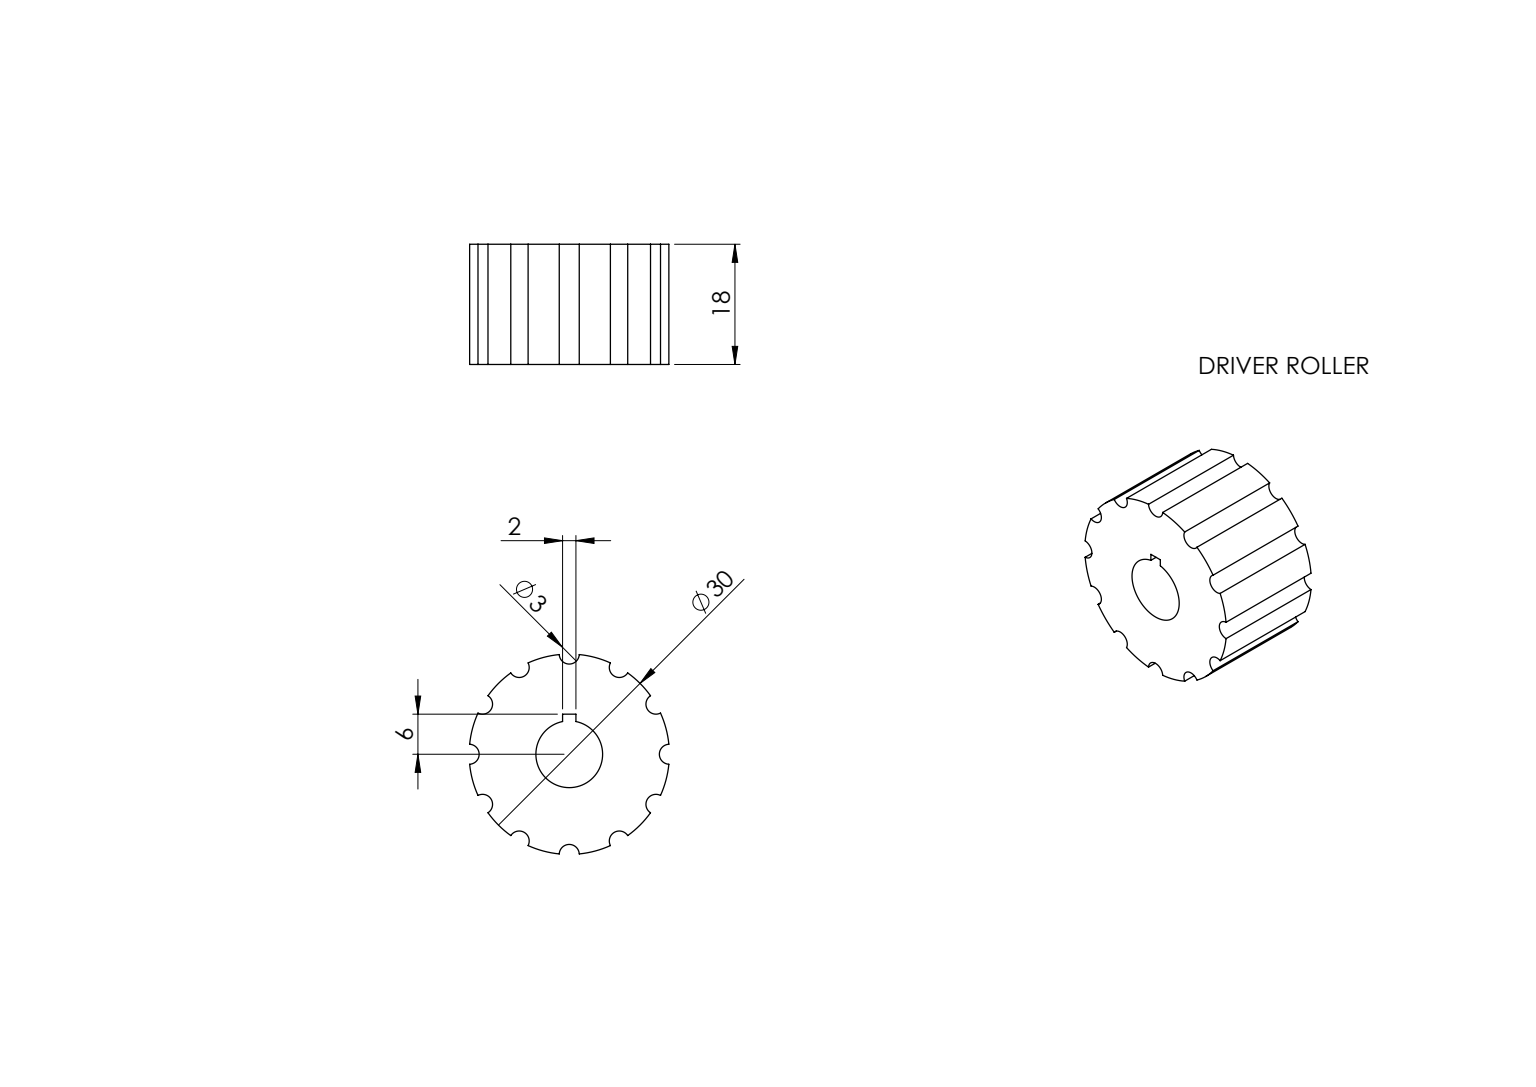
ISO-10303-21;
HEADER;
FILE_DESCRIPTION (('STEP AP214'),
    '1' );
FILE_NAME ('driver roller.step',
    '2026-10-25T07:12:54',
    ( '' ),
    ( '' ),
    'SwSTEP 2.0',
    'SolidWorks 2026',
    '' );
FILE_SCHEMA (( 'AUTOMOTIVE_DESIGN' ));
ENDSEC;

DATA;
#4=DIRECTION ( 'NONE',  ( 0.4999999999999977796, 0.8660254037844398178, 0.000000000000000000 ) ) ;
#12=AXIS2_PLACEMENT_3D ( 'NONE', #12108, #3741, #674 ) ;
#15=CARTESIAN_POINT ( 'NONE',  ( 2.449293598294706513E-15, -35.00000000000000000, 9.000000000000000000 ) ) ;
#19=ADVANCED_FACE ( 'NONE', ( #12392 ), #1035, .T. ) ;
#25=DIRECTION ( 'NONE',  ( -0.000000000000000000, -0.000000000000000000, 1.000000000000000000 ) ) ;
#49=VECTOR ( 'NONE', #8618, 1000.000000000000000 ) ;
#66=CIRCLE ( 'NONE', #7586, 1.500000000000001110 ) ;
#68=LINE ( 'NONE', #4288, #2309 ) ;
#80=CYLINDRICAL_SURFACE ( 'NONE', #13518, 1.500000000000001332 ) ;
#102=DIRECTION ( 'NONE',  ( 1.000000000000000000, 0.000000000000000000, 0.000000000000000000 ) ) ;
#120=ADVANCED_FACE ( 'NONE', ( #5352 ), #80, .F. ) ;
#146=ORIENTED_EDGE ( 'NONE', *, *, #5916, .F. ) ;
#151=DIRECTION ( 'NONE',  ( -0.5000000000000041078, 0.8660254037844362651, 0.000000000000000000 ) ) ;
#153=FACE_OUTER_BOUND ( 'NONE', #3940, .T. ) ;
#154=FACE_OUTER_BOUND ( 'NONE', #10455, .T. ) ;
#193=CYLINDRICAL_SURFACE ( 'NONE', #11066, 15.00000000000000000 ) ;
#198=ORIENTED_EDGE ( 'NONE', *, *, #8722, .T. ) ;
#201=CIRCLE ( 'NONE', #9264, 1.500000000000000222 ) ;
#208=CARTESIAN_POINT ( 'NONE',  ( 2.449293598294706513E-15, -20.00000000000000000, -9.000000000000000000 ) ) ;
#213=ORIENTED_EDGE ( 'NONE', *, *, #10321, .T. ) ;
#227=EDGE_CURVE ( 'NONE', #4104, #6571, #11764, .T. ) ;
#231=VECTOR ( 'NONE', #11750, 1000.000000000000000 ) ;
#239=CARTESIAN_POINT ( 'NONE',  ( 2.449293598294706513E-15, -20.00000000000000000, 9.000000000000000000 ) ) ;
#261=ORIENTED_EDGE ( 'NONE', *, *, #227, .F. ) ;
#265=CARTESIAN_POINT ( 'NONE',  ( 2.449293598294706513E-15, -20.00000000000000000, 9.000000000000000000 ) ) ;
#272=EDGE_CURVE ( 'NONE', #12293, #940, #9194, .T. ) ;
#276=AXIS2_PLACEMENT_3D ( 'NONE', #9355, #962, #6117 ) ;
#277=ORIENTED_EDGE ( 'NONE', *, *, #8722, .F. ) ;
#278=VERTEX_POINT ( 'NONE', #10857 ) ;
#297=ADVANCED_FACE ( 'NONE', ( #10786 ), #7829, .T. ) ;
#299=DIRECTION ( 'NONE',  ( -0.000000000000000000, -0.000000000000000000, -1.000000000000000000 ) ) ;
#310=CIRCLE ( 'NONE', #5415, 1.499999999999999778 ) ;
#317=DIRECTION ( 'NONE',  ( -0.000000000000000000, -0.000000000000000000, 1.000000000000000000 ) ) ;
#318=( NAMED_UNIT ( * ) PLANE_ANGLE_UNIT ( ) SI_UNIT ( $, .RADIAN. ) );
#335=CARTESIAN_POINT ( 'NONE',  ( -11.49038105676659249, -12.50000000000003020, -9.000000000000000000 ) ) ;
#344=ORIENTED_EDGE ( 'NONE', *, *, #1521, .T. ) ;
#348=AXIS2_PLACEMENT_3D ( 'NONE', #13063, #10988, #12044 ) ;
#349=DIRECTION ( 'NONE',  ( 1.000000000000000000, 0.000000000000000000, 0.000000000000000000 ) ) ;
#375=ORIENTED_EDGE ( 'NONE', *, *, #2646, .F. ) ;
#392=ORIENTED_EDGE ( 'NONE', *, *, #1283, .T. ) ;
#402=CARTESIAN_POINT ( 'NONE',  ( 13.67449106481161003, -13.83491329190030861, 9.000000000000000000 ) ) ;
#411=DIRECTION ( 'NONE',  ( -0.000000000000000000, -0.000000000000000000, -1.000000000000000000 ) ) ;
#415=CARTESIAN_POINT ( 'NONE',  ( -6.165086708099452473, -33.67449106481171128, 9.000000000000000000 ) ) ;
#416=CARTESIAN_POINT ( 'NONE',  ( 14.92500000000001492, -21.49812382665770727, -9.000000000000000000 ) ) ;
#430=AXIS2_PLACEMENT_3D ( 'NONE', #5828, #10990, #3471 ) ;
#439=VERTEX_POINT ( 'NONE', #5171 ) ;
#442=CARTESIAN_POINT ( 'NONE',  ( 2.449293598294706513E-15, -20.00000000000000000, 9.000000000000000000 ) ) ;
#453=CIRCLE ( 'NONE', #6010, 5.000000000000000888 ) ;
#476=DIRECTION ( 'NONE',  ( -1.000000000000000000, 0.000000000000000000, 0.000000000000000000 ) ) ;
#478=CARTESIAN_POINT ( 'NONE',  ( -0.9999999999999976685, -20.00000000000000000, 8.999999999999998224 ) ) ;
#483=DIRECTION ( 'NONE',  ( -1.000000000000000000, 0.000000000000000000, 0.000000000000000000 ) ) ;
#487=CARTESIAN_POINT ( 'NONE',  ( 1.000000000000000000, -14.00000000000000000, 8.999999999999998224 ) ) ;
#505=EDGE_CURVE ( 'NONE', #7167, #13447, #11471, .T. ) ;
#535=ORIENTED_EDGE ( 'NONE', *, *, #11080, .F. ) ;
#543=LINE ( 'NONE', #8998, #5245 ) ;
#552=EDGE_LOOP ( 'NONE', ( #11570, #2557, #1287, #708 ) ) ;
#554=CARTESIAN_POINT ( 'NONE',  ( 2.449293598294706513E-15, -20.00000000000000000, 9.000000000000000000 ) ) ;
#561=CARTESIAN_POINT ( 'NONE',  ( -1.498123826657861590, -5.075000000000000178, 9.000000000000000000 ) ) ;
#569=DIRECTION ( 'NONE',  ( 1.000000000000000000, 0.000000000000000000, 0.000000000000000000 ) ) ;
#575=LINE ( 'NONE', #4688, #3098 ) ;
#579=VERTEX_POINT ( 'NONE', #9306 ) ;
#580=ORIENTED_EDGE ( 'NONE', *, *, #12965, .T. ) ;
#582=VERTEX_POINT ( 'NONE', #4050 ) ;
#585=EDGE_CURVE ( 'NONE', #579, #13009, #3012, .T. ) ;
#613=ORIENTED_EDGE ( 'NONE', *, *, #4413, .T. ) ;
#625=DIRECTION ( 'NONE',  ( 1.000000000000000000, 0.000000000000000000, 0.000000000000000000 ) ) ;
#631=CARTESIAN_POINT ( 'NONE',  ( 13.67449106481173615, -26.16508670809940895, 0.000000000000000000 ) ) ;
#636=DIRECTION ( 'NONE',  ( 0.000000000000000000, 0.000000000000000000, -1.000000000000000000 ) ) ;
#655=LINE ( 'NONE', #4833, #12685 ) ;
#672=DIRECTION ( 'NONE',  ( -0.000000000000000000, 0.000000000000000000, 1.000000000000000000 ) ) ;
#674=DIRECTION ( 'NONE',  ( 0.4999999999999977796, 0.8660254037844398178, 0.000000000000000000 ) ) ;
#689=EDGE_CURVE ( 'NONE', #12154, #1369, #11986, .T. ) ;
#694=CARTESIAN_POINT ( 'NONE',  ( -14.92499999999998828, -21.49812382665792754, -9.000000000000000000 ) ) ;
#704=CARTESIAN_POINT ( 'NONE',  ( 6.165086708099353885, -6.325508935188239867, -9.000000000000000000 ) ) ;
#708=ORIENTED_EDGE ( 'NONE', *, *, #3659, .T. ) ;
#744=CYLINDRICAL_SURFACE ( 'NONE', #7474, 1.500000000000001332 ) ;
#746=AXIS2_PLACEMENT_3D ( 'NONE', #10700, #7661, #9662 ) ;
#758=EDGE_LOOP ( 'NONE', ( #6496, #10523, #13430, #10250 ) ) ;
#761=ORIENTED_EDGE ( 'NONE', *, *, #9825, .T. ) ;
#762=EDGE_LOOP ( 'NONE', ( #12304, #11458, #12169, #8097 ) ) ;
#769=EDGE_CURVE ( 'NONE', #9673, #2278, #201, .T. ) ;
#772=CARTESIAN_POINT ( 'NONE',  ( -12.99038105676654453, -27.50000000000006040, -9.000000000000000000 ) ) ;
#796=ORIENTED_EDGE ( 'NONE', *, *, #2151, .F. ) ;
#803=CARTESIAN_POINT ( 'NONE',  ( -13.49999999999999467, -20.00000000000005329, 9.000000000000000000 ) ) ;
#807=ORIENTED_EDGE ( 'NONE', *, *, #11080, .T. ) ;
#812=CARTESIAN_POINT ( 'NONE',  ( 8.759913291900563337, -32.17636723815374467, 9.000000000000000000 ) ) ;
#821=ORIENTED_EDGE ( 'NONE', *, *, #11191, .T. ) ;
#825=DIRECTION ( 'NONE',  ( -0.000000000000000000, -0.000000000000000000, 1.000000000000000000 ) ) ;
#843=AXIS2_PLACEMENT_3D ( 'NONE', #13504, #4053, #8278 ) ;
#846=EDGE_CURVE ( 'NONE', #7079, #13382, #12319, .T. ) ;
#848=AXIS2_PLACEMENT_3D ( 'NONE', #6811, #5853, #7015 ) ;
#850=AXIS2_PLACEMENT_3D ( 'NONE', #4188, #4255, #986 ) ;
#881=ORIENTED_EDGE ( 'NONE', *, *, #13242, .T. ) ;
#887=CYLINDRICAL_SURFACE ( 'NONE', #10653, 1.500000000000000444 ) ;
#895=VECTOR ( 'NONE', #4344, 1000.000000000000000 ) ;
#896=ORIENTED_EDGE ( 'NONE', *, *, #12447, .T. ) ;
#904=AXIS2_PLACEMENT_3D ( 'NONE', #10254, #2791, #7010 ) ;
#913=CARTESIAN_POINT ( 'NONE',  ( -1.000000000000000000, -14.00000000000000000, 8.999999999999998224 ) ) ;
#921=CIRCLE ( 'NONE', #4467, 1.500000000000000666 ) ;
#925=CARTESIAN_POINT ( 'NONE',  ( 2.449293598294706513E-15, -20.00000000000000000, -9.000000000000000000 ) ) ;
#927=CARTESIAN_POINT ( 'NONE',  ( 2.449293598294706513E-15, -20.00000000000000000, -8.999999999999998224 ) ) ;
#929=DIRECTION ( 'NONE',  ( -4.082155997157844188E-16, 1.000000000000000000, 0.000000000000000000 ) ) ;
#935=AXIS2_PLACEMENT_3D ( 'NONE', #208, #4428, #11687 ) ;
#940=VERTEX_POINT ( 'NONE', #3983 ) ;
#947=DIRECTION ( 'NONE',  ( -0.8660254037844412611, 0.4999999999999956146, 0.000000000000000000 ) ) ;
#951=ORIENTED_EDGE ( 'NONE', *, *, #9608, .T. ) ;
#961=MANIFOLD_SOLID_BREP ( 'Cavity1', #5391 ) ;
#962=DIRECTION ( 'NONE',  ( 0.000000000000000000, 0.000000000000000000, 1.000000000000000000 ) ) ;
#965=AXIS2_PLACEMENT_3D ( 'NONE', #4001, #12570, #10361 ) ;
#980=DIRECTION ( 'NONE',  ( 0.000000000000000000, -0.000000000000000000, 1.000000000000000000 ) ) ;
#986=DIRECTION ( 'NONE',  ( 1.000000000000000000, 0.000000000000000000, 0.000000000000000000 ) ) ;
#996=CARTESIAN_POINT ( 'NONE',  ( 2.449293598294706513E-15, -20.00000000000000000, 9.000000000000000000 ) ) ;
#998=CARTESIAN_POINT ( 'NONE',  ( -6.165086708099547508, -6.325508935188330462, 9.000000000000000000 ) ) ;
#1033=ORIENTED_EDGE ( 'NONE', *, *, #12965, .F. ) ;
#1034=ORIENTED_EDGE ( 'NONE', *, *, #11991, .F. ) ;
#1035=CYLINDRICAL_SURFACE ( 'NONE', #7896, 15.00000000000000000 ) ;
#1061=CARTESIAN_POINT ( 'NONE',  ( 2.449293598294706513E-15, -20.00000000000000000, 9.000000000000000000 ) ) ;
#1074=DIRECTION ( 'NONE',  ( 0.000000000000000000, 0.000000000000000000, 1.000000000000000000 ) ) ;
#1095=ADVANCED_FACE ( 'NONE', ( #9833 ), #7627, .T. ) ;
#1097=ADVANCED_FACE ( 'NONE', ( #154 ), #12997, .T. ) ;
#1100=ORIENTED_EDGE ( 'NONE', *, *, #4158, .F. ) ;
#1104=DIRECTION ( 'NONE',  ( 0.000000000000000000, 0.000000000000000000, 1.000000000000000000 ) ) ;
#1121=AXIS2_PLACEMENT_3D ( 'NONE', #4108, #13625, #12728 ) ;
#1145=AXIS2_PLACEMENT_3D ( 'NONE', #11029, #10129, #4890 ) ;
#1149=CIRCLE ( 'NONE', #9121, 15.00000000000000000 ) ;
#1153=DIRECTION ( 'NONE',  ( 0.000000000000000000, 0.000000000000000000, 1.000000000000000000 ) ) ;
#1169=ORIENTED_EDGE ( 'NONE', *, *, #5857, .F. ) ;
#1189=VECTOR ( 'NONE', #11314, 1000.000000000000000 ) ;
#1192=DIRECTION ( 'NONE',  ( 1.000000000000000000, 0.000000000000000000, 0.000000000000000000 ) ) ;
#1220=EDGE_CURVE ( 'NONE', #12388, #4959, #11203, .T. ) ;
#1223=VERTEX_POINT ( 'NONE', #5831 ) ;
#1234=ORIENTED_EDGE ( 'NONE', *, *, #13277, .T. ) ;
#1247=EDGE_LOOP ( 'NONE', ( #12529, #10799, #10589, #5654, #761, #4432 ) ) ;
#1249=ORIENTED_EDGE ( 'NONE', *, *, #9161, .F. ) ;
#1250=LINE ( 'NONE', #6287, #3951 ) ;
#1262=DIRECTION ( 'NONE',  ( 0.000000000000000000, 0.000000000000000000, 1.000000000000000000 ) ) ;
#1273=FILL_AREA_STYLE_COLOUR ( '', #1315 ) ;
#1282=DIRECTION ( 'NONE',  ( 0.8660254037844381525, 0.5000000000000009992, 0.000000000000000000 ) ) ;
#1283=EDGE_CURVE ( 'NONE', #10723, #6266, #543, .T. ) ;
#1287=ORIENTED_EDGE ( 'NONE', *, *, #1283, .F. ) ;
#1302=VERTEX_POINT ( 'NONE', #6927 ) ;
#1312=CYLINDRICAL_SURFACE ( 'NONE', #5790, 15.00000000000000000 ) ;
#1315=COLOUR_RGB ( '',0.8941176470588234615, 0.8941176470588234615, 0.8941176470588234615 ) ;
#1353=CARTESIAN_POINT ( 'NONE',  ( 2.449293598294706513E-15, -20.00000000000000000, 9.000000000000000000 ) ) ;
#1369=VERTEX_POINT ( 'NONE', #9546 ) ;
#1389=CARTESIAN_POINT ( 'NONE',  ( 6.165086708099646984, -33.67449106481162602, 0.000000000000000000 ) ) ;
#1403=APPLICATION_CONTEXT ( 'automotive_design' ) ;
#1407=DIRECTION ( 'NONE',  ( 1.000000000000000000, 0.000000000000000000, 0.000000000000000000 ) ) ;
#1419=VECTOR ( 'NONE', #636, 1000.000000000000000 ) ;
#1439=ORIENTED_EDGE ( 'NONE', *, *, #1549, .F. ) ;
#1459=PRODUCT_DEFINITION_SHAPE ( 'NONE', 'NONE',  #12493 ) ;
#1460=LINE ( 'NONE', #5706, #13111 ) ;
#1466=DIRECTION ( 'NONE',  ( -1.000000000000000000, 0.000000000000000000, 0.000000000000000000 ) ) ;
#1474=DIRECTION ( 'NONE',  ( -4.082155997157844188E-16, 1.000000000000000000, 0.000000000000000000 ) ) ;
#1508=VERTEX_POINT ( 'NONE', #6256 ) ;
#1510=DIRECTION ( 'NONE',  ( 1.000000000000000000, 0.000000000000000000, 0.000000000000000000 ) ) ;
#1513=DIRECTION ( 'NONE',  ( 1.000000000000000000, 0.000000000000000000, 0.000000000000000000 ) ) ;
#1515=DIRECTION ( 'NONE',  ( -1.000000000000000000, 0.000000000000000000, 0.000000000000000000 ) ) ;
#1521=EDGE_CURVE ( 'NONE', #4218, #582, #5409, .T. ) ;
#1530=CARTESIAN_POINT ( 'NONE',  ( 7.499999999999834799, -7.009618943233325794, -9.000000000000000000 ) ) ;
#1548=CARTESIAN_POINT ( 'NONE',  ( 12.17636723815371447, -11.24008670809939581, 9.000000000000000000 ) ) ;
#1549=EDGE_CURVE ( 'NONE', #6599, #6478, #2894, .T. ) ;
#1582=DIRECTION ( 'NONE',  ( -0.8660254037844412611, 0.4999999999999956146, 0.000000000000000000 ) ) ;
#1606=DIRECTION ( 'NONE',  ( 1.000000000000000000, 0.000000000000000000, 0.000000000000000000 ) ) ;
#1607=ORIENTED_EDGE ( 'NONE', *, *, #769, .T. ) ;
#1608=UNCERTAINTY_MEASURE_WITH_UNIT (LENGTH_MEASURE( 1.000000000000000082E-05 ), #10444, 'distance_accuracy_value', 'NONE');
#1622=CARTESIAN_POINT ( 'NONE',  ( -1.000000000000000000, -14.00000000000000000, 8.999999999999998224 ) ) ;
#1638=CIRCLE ( 'NONE', #6092, 15.00000000000000000 ) ;
#1645=ORIENTED_EDGE ( 'NONE', *, *, #7550, .F. ) ;
#1648=DIRECTION ( 'NONE',  ( 0.8660254037844381525, 0.5000000000000009992, 0.000000000000000000 ) ) ;
#1650=EDGE_CURVE ( 'NONE', #4030, #12154, #7403, .T. ) ;
#1665=DIRECTION ( 'NONE',  ( 0.8660254037844381525, 0.5000000000000009992, 0.000000000000000000 ) ) ;
#1667=DIRECTION ( 'NONE',  ( -0.5000000000000041078, 0.8660254037844362651, 0.000000000000000000 ) ) ;
#1680=ORIENTED_EDGE ( 'NONE', *, *, #8779, .F. ) ;
#1740=DIRECTION ( 'NONE',  ( 1.040834085586083310E-14, -1.000000000000000000, 0.000000000000000000 ) ) ;
#1755=ORIENTED_EDGE ( 'NONE', *, *, #13336, .F. ) ;
#1758=DIRECTION ( 'NONE',  ( -9.858538378746663627E-23, 5.031452844637890958E-23, -1.000000000000000000 ) ) ;
#1774=EDGE_LOOP ( 'NONE', ( #5944, #2961, #9843, #12955 ) ) ;
#1780=VECTOR ( 'NONE', #9908, 1000.000000000000000 ) ;
#1792=CYLINDRICAL_SURFACE ( 'NONE', #7254, 15.00000000000000000 ) ;
#1813=CARTESIAN_POINT ( 'NONE',  ( -14.92499999999998828, -21.49812382665791688, 9.000000000000000000 ) ) ;
#1843=VERTEX_POINT ( 'NONE', #2389 ) ;
#1857=VERTEX_POINT ( 'NONE', #5521 ) ;
#1867=CARTESIAN_POINT ( 'NONE',  ( 1.498123826657866475, -5.075000000000000178, -9.000000000000000000 ) ) ;
#1879=EDGE_LOOP ( 'NONE', ( #8930, #10856, #8607, #6643 ) ) ;
#1881=EDGE_LOOP ( 'NONE', ( #12271, #2264, #5006, #277 ) ) ;
#1898=ORIENTED_EDGE ( 'NONE', *, *, #13606, .F. ) ;
#1900=AXIS2_PLACEMENT_3D ( 'NONE', #913, #9299, #8403 ) ;
#1926=ORIENTED_EDGE ( 'NONE', *, *, #13606, .T. ) ;
#1927=EDGE_LOOP ( 'NONE', ( #10839, #7588, #9235, #5962 ) ) ;
#1928=ORIENTED_EDGE ( 'NONE', *, *, #12695, .F. ) ;
#1943=EDGE_LOOP ( 'NONE', ( #3043, #4233, #2144, #2017 ) ) ;
#1951=CARTESIAN_POINT ( 'NONE',  ( 2.449293598294706513E-15, -20.00000000000000000, 9.000000000000000000 ) ) ;
#1955=CIRCLE ( 'NONE', #3499, 15.00000000000000000 ) ;
#1960=CARTESIAN_POINT ( 'NONE',  ( 2.449293598294706513E-15, -20.00000000000000000, 15.00000000000000355 ) ) ;
#1968=CIRCLE ( 'NONE', #5948, 1.500000000000000222 ) ;
#1969=ORIENTED_EDGE ( 'NONE', *, *, #13348, .F. ) ;
#1975=DIRECTION ( 'NONE',  ( 1.000000000000000000, -6.938893903907227392E-16, 0.000000000000000000 ) ) ;
#1992=DIRECTION ( 'NONE',  ( 0.000000000000000000, -0.000000000000000000, 1.000000000000000000 ) ) ;
#2006=FACE_OUTER_BOUND ( 'NONE', #758, .T. ) ;
#2017=ORIENTED_EDGE ( 'NONE', *, *, #7591, .T. ) ;
#2023=AXIS2_PLACEMENT_3D ( 'NONE', #1951, #6398, #6196 ) ;
#2025=AXIS2_PLACEMENT_3D ( 'NONE', #7469, #1153, #1282 ) ;
#2038=EDGE_LOOP ( 'NONE', ( #1928, #7008, #535, #8066, #1169, #11779 ) ) ;
#2054=EDGE_LOOP ( 'NONE', ( #807, #5754, #11148, #12724 ) ) ;
#2055=FACE_OUTER_BOUND ( 'NONE', #4086, .T. ) ;
#2065=CARTESIAN_POINT ( 'NONE',  ( 15.00000000000000355, -19.99999999999984368, -9.000000000000000000 ) ) ;
#2067=VERTEX_POINT ( 'NONE', #10893 ) ;
#2078=AXIS2_PLACEMENT_3D ( 'NONE', #6069, #8129, #1606 ) ;
#2080=ORIENTED_EDGE ( 'NONE', *, *, #227, .T. ) ;
#2087=DIRECTION ( 'NONE',  ( 1.000000000000000000, 0.000000000000000000, 0.000000000000000000 ) ) ;
#2091=LINE ( 'NONE', #6336, #7295 ) ;
#2107=DIRECTION ( 'NONE',  ( -1.000000000000000000, 0.000000000000000000, 0.000000000000000000 ) ) ;
#2116=VERTEX_POINT ( 'NONE', #1548 ) ;
#2144=ORIENTED_EDGE ( 'NONE', *, *, #4008, .T. ) ;
#2149=CARTESIAN_POINT ( 'NONE',  ( 2.449293598294706513E-15, -20.00000000000000000, 9.000000000000000000 ) ) ;
#2151=EDGE_CURVE ( 'NONE', #10268, #4104, #8551, .T. ) ;
#2175=DIRECTION ( 'NONE',  ( 1.000000000000000000, 0.000000000000000000, -0.000000000000000000 ) ) ;
#2202=CARTESIAN_POINT ( 'NONE',  ( 8.759913291900311094, -7.823632761846075923, 0.000000000000000000 ) ) ;
#2239=ADVANCED_FACE ( 'NONE', ( #5510 ), #12815, .F. ) ;
#2264=ORIENTED_EDGE ( 'NONE', *, *, #1549, .T. ) ;
#2278=VERTEX_POINT ( 'NONE', #6551 ) ;
#2286=DIRECTION ( 'NONE',  ( -1.000000000000000000, 0.000000000000000000, 0.000000000000000000 ) ) ;
#2306=CARTESIAN_POINT ( 'NONE',  ( 2.449293598294706513E-15, -20.00000000000000000, -9.000000000000000000 ) ) ;
#2309=VECTOR ( 'NONE', #4488, 1000.000000000000000 ) ;
#2320=ORIENTED_EDGE ( 'NONE', *, *, #8072, .F. ) ;
#2336=LINE ( 'NONE', #5536, #3110 ) ;
#2342=CARTESIAN_POINT ( 'NONE',  ( -12.99038105676659427, -12.50000000000003020, 9.000000000000000000 ) ) ;
#2345=ORIENTED_EDGE ( 'NONE', *, *, #3394, .F. ) ;
#2362=EDGE_CURVE ( 'NONE', #439, #6571, #10852, .T. ) ;
#2381=ORIENTED_EDGE ( 'NONE', *, *, #4240, .T. ) ;
#2384=VERTEX_POINT ( 'NONE', #561 ) ;
#2389=CARTESIAN_POINT ( 'NONE',  ( 13.67449106481174148, -26.16508670809939829, -9.000000000000000000 ) ) ;
#2393=LINE ( 'NONE', #12768, #11694 ) ;
#2401=ADVANCED_FACE ( 'NONE', ( #2725 ), #7917, .F. ) ;
#2418=DIRECTION ( 'NONE',  ( 0.000000000000000000, 0.000000000000000000, 1.000000000000000000 ) ) ;
#2428=CARTESIAN_POINT ( 'NONE',  ( 2.449293598294706513E-15, -20.00000000000000000, 9.000000000000000000 ) ) ;
#2433=EDGE_CURVE ( 'NONE', #579, #12390, #11836, .T. ) ;
#2438=DIRECTION ( 'NONE',  ( 1.000000000000000000, 0.000000000000000000, 0.000000000000000000 ) ) ;
#2443=DIRECTION ( 'NONE',  ( -0.000000000000000000, -0.000000000000000000, -1.000000000000000000 ) ) ;
#2444=DIRECTION ( 'NONE',  ( 0.4999999999999977796, 0.8660254037844398178, 0.000000000000000000 ) ) ;
#2452=ORIENTED_EDGE ( 'NONE', *, *, #7450, .F. ) ;
#2485=AXIS2_PLACEMENT_3D ( 'NONE', #12752, #6985, #10884 ) ;
#2503=ORIENTED_EDGE ( 'NONE', *, *, #12212, .F. ) ;
#2522=ORIENTED_EDGE ( 'NONE', *, *, #11531, .F. ) ;
#2555=AXIS2_PLACEMENT_3D ( 'NONE', #1960, #6203, #12733 ) ;
#2557=ORIENTED_EDGE ( 'NONE', *, *, #8401, .F. ) ;
#2563=CYLINDRICAL_SURFACE ( 'NONE', #6455, 1.500000000000001332 ) ;
#2573=ORIENTED_EDGE ( 'NONE', *, *, #6544, .T. ) ;
#2577=EDGE_CURVE ( 'NONE', #7202, #5253, #10068, .T. ) ;
#2588=VERTEX_POINT ( 'NONE', #3966 ) ;
#2600=ADVANCED_FACE ( 'NONE', ( #10261 ), #4179, .F. ) ;
#2605=ADVANCED_FACE ( 'NONE', ( #13493 ), #11296, .F. ) ;
#2627=DIRECTION ( 'NONE',  ( -0.000000000000000000, -0.000000000000000000, -1.000000000000000000 ) ) ;
#2631=CIRCLE ( 'NONE', #11019, 1.500000000000000666 ) ;
#2646=EDGE_CURVE ( 'NONE', #5253, #4470, #13631, .T. ) ;
#2648=DIRECTION ( 'NONE',  ( -4.082155997157844188E-16, 1.000000000000000000, 0.000000000000000000 ) ) ;
#2649=CARTESIAN_POINT ( 'NONE',  ( 2.449293598294706513E-15, -20.00000000000000000, -9.000000000000000000 ) ) ;
#2670=FACE_OUTER_BOUND ( 'NONE', #8845, .T. ) ;
#2712=ORIENTED_EDGE ( 'NONE', *, *, #9792, .T. ) ;
#2725=FACE_OUTER_BOUND ( 'NONE', #13498, .T. ) ;
#2733=ORIENTED_EDGE ( 'NONE', *, *, #9161, .T. ) ;
#2736=ADVANCED_FACE ( 'NONE', ( #3005 ), #11436, .F. ) ;
#2741=AXIS2_PLACEMENT_3D ( 'NONE', #7558, #1104, #2087 ) ;
#2773=CARTESIAN_POINT ( 'NONE',  ( 2.449293598294706513E-15, -20.00000000000000000, 9.000000000000000000 ) ) ;
#2791=DIRECTION ( 'NONE',  ( 0.000000000000000000, -0.000000000000000000, 1.000000000000000000 ) ) ;
#2807=VERTEX_POINT ( 'NONE', #7498 ) ;
#2847=CIRCLE ( 'NONE', #10121, 1.500000000000001554 ) ;
#2857=CARTESIAN_POINT ( 'NONE',  ( -4.999999999999998224, -20.00000000000000000, -8.999999999999998224 ) ) ;
#2864=DIRECTION ( 'NONE',  ( 1.000000000000000000, 0.000000000000000000, 0.000000000000000000 ) ) ;
#2875=CARTESIAN_POINT ( 'NONE',  ( 2.449293598294706513E-15, -20.00000000000000000, -8.999999999999998224 ) ) ;
#2877=AXIS2_PLACEMENT_3D ( 'NONE', #996, #6356, #5107 ) ;
#2894=LINE ( 'NONE', #4072, #6089 ) ;
#2913=EDGE_CURVE ( 'NONE', #7674, #940, #1149, .T. ) ;
#2918=VECTOR ( 'NONE', #6042, 1000.000000000000000 ) ;
#2926=PRODUCT_DEFINITION_CONTEXT ( 'detailed design', #1403, 'design' ) ;
#2938=CARTESIAN_POINT ( 'NONE',  ( -6.000000000000013323, -7.009618943233427935, -9.000000000000000000 ) ) ;
#2956=CARTESIAN_POINT ( 'NONE',  ( 2.449293598294706513E-15, -20.00000000000000000, -9.000000000000000000 ) ) ;
#2961=ORIENTED_EDGE ( 'NONE', *, *, #585, .F. ) ;
#2965=CIRCLE ( 'NONE', #12043, 5.000000000000000888 ) ;
#2983=DIRECTION ( 'NONE',  ( 0.000000000000000000, 0.000000000000000000, 1.000000000000000000 ) ) ;
#2996=VERTEX_POINT ( 'NONE', #416 ) ;
#2998=DIRECTION ( 'NONE',  ( 1.040834085586083310E-14, -1.000000000000000000, 0.000000000000000000 ) ) ;
#3000=SHAPE_DEFINITION_REPRESENTATION ( #1459, #10521 ) ;
#3004=CARTESIAN_POINT ( 'NONE',  ( -1.000000000000000000, -14.00000000000000000, 8.999999999999998224 ) ) ;
#3005=FACE_OUTER_BOUND ( 'NONE', #762, .T. ) ;
#3012=LINE ( 'NONE', #5564, #7937 ) ;
#3013=ORIENTED_EDGE ( 'NONE', *, *, #8473, .F. ) ;
#3028=ORIENTED_EDGE ( 'NONE', *, *, #4761, .F. ) ;
#3035=DIRECTION ( 'NONE',  ( 1.000000000000000000, 0.000000000000000000, 0.000000000000000000 ) ) ;
#3043=ORIENTED_EDGE ( 'NONE', *, *, #2433, .F. ) ;
#3081=ORIENTED_EDGE ( 'NONE', *, *, #272, .T. ) ;
#3098=VECTOR ( 'NONE', #4821, 1000.000000000000000 ) ;
#3100=DIRECTION ( 'NONE',  ( -0.000000000000000000, 0.000000000000000000, 1.000000000000000000 ) ) ;
#3110=VECTOR ( 'NONE', #6711, 1000.000000000000000 ) ;
#3133=AXIS2_PLACEMENT_3D ( 'NONE', #7644, #299, #4526 ) ;
#3148=AXIS2_PLACEMENT_3D ( 'NONE', #5589, #10445, #3185 ) ;
#3171=CARTESIAN_POINT ( 'NONE',  ( 6.165086708099646984, -33.67449106481162602, 9.000000000000000000 ) ) ;
#3185=DIRECTION ( 'NONE',  ( 1.000000000000000000, 0.000000000000000000, 0.000000000000000000 ) ) ;
#3198=ORIENTED_EDGE ( 'NONE', *, *, #7704, .T. ) ;
#3208=EDGE_CURVE ( 'NONE', #2278, #4659, #3592, .T. ) ;
#3211=DIRECTION ( 'NONE',  ( 1.000000000000000000, 0.000000000000000000, 0.000000000000000000 ) ) ;
#3222=DIRECTION ( 'NONE',  ( 0.000000000000000000, 0.000000000000000000, 1.000000000000000000 ) ) ;
#3226=CARTESIAN_POINT ( 'NONE',  ( 2.449293598294706513E-15, -20.00000000000000000, 9.000000000000000000 ) ) ;
#3278=LINE ( 'NONE', #11244, #1189 ) ;
#3284=EDGE_CURVE ( 'NONE', #11391, #6039, #12639, .T. ) ;
#3286=DIRECTION ( 'NONE',  ( 1.000000000000000000, 0.000000000000000000, 0.000000000000000000 ) ) ;
#3287=CIRCLE ( 'NONE', #11893, 15.00000000000000000 ) ;
#3292=DIRECTION ( 'NONE',  ( 0.000000000000000000, 0.000000000000000000, 1.000000000000000000 ) ) ;
#3297=AXIS2_PLACEMENT_3D ( 'NONE', #4668, #9721, #2444 ) ;
#3303=DIRECTION ( 'NONE',  ( 0.000000000000000000, 0.000000000000000000, 1.000000000000000000 ) ) ;
#3315=AXIS2_PLACEMENT_3D ( 'NONE', #3226, #5037, #2107 ) ;
#3317=ORIENTED_EDGE ( 'NONE', *, *, #11597, .F. ) ;
#3319=CARTESIAN_POINT ( 'NONE',  ( 8.759913291900572219, -32.17636723815373756, -9.000000000000000000 ) ) ;
#3332=VECTOR ( 'NONE', #10774, 1000.000000000000000 ) ;
#3343=DIRECTION ( 'NONE',  ( 0.000000000000000000, 0.000000000000000000, 1.000000000000000000 ) ) ;
#3364=AXIS2_PLACEMENT_3D ( 'NONE', #7013, #11224, #4879 ) ;
#3368=ORIENTED_EDGE ( 'NONE', *, *, #13564, .T. ) ;
#3372=( NAMED_UNIT ( * ) SI_UNIT ( $, .STERADIAN. ) SOLID_ANGLE_UNIT ( ) );
#3383=ORIENTED_EDGE ( 'NONE', *, *, #3659, .F. ) ;
#3394=EDGE_CURVE ( 'NONE', #10160, #4300, #8451, .T. ) ;
#3422=FACE_OUTER_BOUND ( 'NONE', #8151, .T. ) ;
#3440=( NAMED_UNIT ( * ) PLANE_ANGLE_UNIT ( ) SI_UNIT ( $, .RADIAN. ) );
#3451=ORIENTED_EDGE ( 'NONE', *, *, #10943, .F. ) ;
#3455=CARTESIAN_POINT ( 'NONE',  ( -6.165086708099547508, -6.325508935188330462, 0.000000000000000000 ) ) ;
#3471=DIRECTION ( 'NONE',  ( 1.000000000000000000, 0.000000000000000000, 0.000000000000000000 ) ) ;
#3483=ORIENTED_EDGE ( 'NONE', *, *, #3985, .T. ) ;
#3498=VERTEX_POINT ( 'NONE', #402 ) ;
#3499=AXIS2_PLACEMENT_3D ( 'NONE', #442, #8962, #569 ) ;
#3521=ORIENTED_EDGE ( 'NONE', *, *, #2151, .T. ) ;
#3535=EDGE_LOOP ( 'NONE', ( #6737, #5076, #12595, #2320 ) ) ;
#3555=LINE ( 'NONE', #1389, #1780 ) ;
#3570=VECTOR ( 'NONE', #13562, 1000.000000000000000 ) ;
#3574=DIRECTION ( 'NONE',  ( -0.000000000000000000, -0.000000000000000000, 1.000000000000000000 ) ) ;
#3577=LINE ( 'NONE', #7866, #5778 ) ;
#3592=CIRCLE ( 'NONE', #276, 1.500000000000000222 ) ;
#3603=ORIENTED_EDGE ( 'NONE', *, *, #8717, .T. ) ;
#3612=FACE_OUTER_BOUND ( 'NONE', #1927, .T. ) ;
#3632=DIRECTION ( 'NONE',  ( 0.000000000000000000, 0.000000000000000000, 1.000000000000000000 ) ) ;
#3643=CARTESIAN_POINT ( 'NONE',  ( -12.99038105676654453, -27.50000000000006040, -9.000000000000000000 ) ) ;
#3654=ORIENTED_EDGE ( 'NONE', *, *, #3284, .T. ) ;
#3658=CYLINDRICAL_SURFACE ( 'NONE', #6835, 1.500000000000000444 ) ;
#3659=EDGE_CURVE ( 'NONE', #10723, #10160, #66, .T. ) ;
#3673=VERTEX_POINT ( 'NONE', #3936 ) ;
#3704=LINE ( 'NONE', #3774, #1419 ) ;
#3706=DIRECTION ( 'NONE',  ( 1.000000000000000000, 0.000000000000000000, 0.000000000000000000 ) ) ;
#3714=ORIENTED_EDGE ( 'NONE', *, *, #9959, .F. ) ;
#3717=ORIENTED_EDGE ( 'NONE', *, *, #12089, .T. ) ;
#3720=DIRECTION ( 'NONE',  ( 1.000000000000000000, 0.000000000000000000, 0.000000000000000000 ) ) ;
#3733=ORIENTED_EDGE ( 'NONE', *, *, #9061, .T. ) ;
#3741=DIRECTION ( 'NONE',  ( 0.000000000000000000, 0.000000000000000000, 1.000000000000000000 ) ) ;
#3743=DIRECTION ( 'NONE',  ( 0.000000000000000000, 0.000000000000000000, -1.000000000000000000 ) ) ;
#3767=CARTESIAN_POINT ( 'NONE',  ( 2.449293598294706513E-15, -20.00000000000000000, -9.000000000000000000 ) ) ;
#3774=CARTESIAN_POINT ( 'NONE',  ( -1.498123826657861590, -5.075000000000000178, 0.000000000000000000 ) ) ;
#3794=ADVANCED_FACE ( 'NONE', ( #4334 ), #8555, .T. ) ;
#3810=LINE ( 'NONE', #4783, #6585 ) ;
#3840=EDGE_LOOP ( 'NONE', ( #3714, #580, #4433, #6988 ) ) ;
#3850=CARTESIAN_POINT ( 'NONE',  ( -14.92500000000000249, -18.50187617334218970, 9.000000000000000000 ) ) ;
#3862=CIRCLE ( 'NONE', #5635, 15.00000000000000000 ) ;
#3873=EDGE_LOOP ( 'NONE', ( #7774, #613, #4627, #375 ) ) ;
#3891=VERTEX_POINT ( 'NONE', #5717 ) ;
#3915=CARTESIAN_POINT ( 'NONE',  ( -12.99038105676659427, -12.50000000000003020, -9.000000000000000000 ) ) ;
#3929=FACE_OUTER_BOUND ( 'NONE', #8624, .T. ) ;
#3933=EDGE_CURVE ( 'NONE', #6494, #8472, #13323, .T. ) ;
#3936=CARTESIAN_POINT ( 'NONE',  ( 5.000000000000003553, -20.00000000000000000, 9.000000000000000000 ) ) ;
#3940=EDGE_LOOP ( 'NONE', ( #1034, #2573, #4866, #344 ) ) ;
#3943=CIRCLE ( 'NONE', #7484, 5.000000000000000888 ) ;
#3946=CARTESIAN_POINT ( 'NONE',  ( 12.17636723815389566, -28.75991329190035373, 9.000000000000000000 ) ) ;
#3951=VECTOR ( 'NONE', #7706, 1000.000000000000000 ) ;
#3959=ORIENTED_EDGE ( 'NONE', *, *, #7633, .F. ) ;
#3961=CARTESIAN_POINT ( 'NONE',  ( 15.00000000000000355, -19.99999999999984368, -9.000000000000000000 ) ) ;
#3966=CARTESIAN_POINT ( 'NONE',  ( -8.759913291900394583, -32.17636723815387256, 9.000000000000000000 ) ) ;
#3983=CARTESIAN_POINT ( 'NONE',  ( -13.67449106481164733, -26.16508670809959725, -9.000000000000000000 ) ) ;
#3985=EDGE_CURVE ( 'NONE', #1302, #4555, #12462, .T. ) ;
#4001=CARTESIAN_POINT ( 'NONE',  ( 2.449293598294706513E-15, -20.00000000000000000, -9.000000000000000000 ) ) ;
#4008=EDGE_CURVE ( 'NONE', #13009, #10020, #6305, .T. ) ;
#4030=VERTEX_POINT ( 'NONE', #11160 ) ;
#4036=DIRECTION ( 'NONE',  ( 0.8660254037844450359, -0.4999999999999888423, 0.000000000000000000 ) ) ;
#4044=LINE ( 'NONE', #2938, #6896 ) ;
#4047=DIRECTION ( 'NONE',  ( -0.000000000000000000, -0.000000000000000000, -1.000000000000000000 ) ) ;
#4048=ORIENTED_EDGE ( 'NONE', *, *, #4791, .T. ) ;
#4050=CARTESIAN_POINT ( 'NONE',  ( 8.759913291900311094, -7.823632761846075923, 9.000000000000000000 ) ) ;
#4053=DIRECTION ( 'NONE',  ( 0.000000000000000000, 0.000000000000000000, 1.000000000000000000 ) ) ;
#4071=CARTESIAN_POINT ( 'NONE',  ( 12.99038105676665289, -27.49999999999988276, 9.000000000000000000 ) ) ;
#4072=CARTESIAN_POINT ( 'NONE',  ( -5.999999999999922728, -32.99038105676662269, -9.000000000000000000 ) ) ;
#4082=AXIS2_PLACEMENT_3D ( 'NONE', #8331, #5084, #2998 ) ;
#4086=EDGE_LOOP ( 'NONE', ( #9172, #12991, #12937, #1607 ) ) ;
#4092=DIRECTION ( 'NONE',  ( 0.000000000000000000, -0.000000000000000000, 1.000000000000000000 ) ) ;
#4104=VERTEX_POINT ( 'NONE', #704 ) ;
#4108=CARTESIAN_POINT ( 'NONE',  ( 2.449293598294706513E-15, -20.00000000000000000, 9.000000000000000000 ) ) ;
#4121=ORIENTED_EDGE ( 'NONE', *, *, #4329, .F. ) ;
#4124=AXIS2_PLACEMENT_3D ( 'NONE', #4738, #5917, #6810 ) ;
#4140=CARTESIAN_POINT ( 'NONE',  ( -11.49038105676654453, -27.50000000000006040, -9.000000000000000000 ) ) ;
#4151=DIRECTION ( 'NONE',  ( 0.5000000000000103251, -0.8660254037844327124, 0.000000000000000000 ) ) ;
#4158=EDGE_CURVE ( 'NONE', #1302, #1843, #10119, .T. ) ;
#4174=CIRCLE ( 'NONE', #843, 1.500000000000000666 ) ;
#4179=CYLINDRICAL_SURFACE ( 'NONE', #13597, 1.500000000000001332 ) ;
#4188=CARTESIAN_POINT ( 'NONE',  ( 2.449293598294706513E-15, -20.00000000000000000, -8.999999999999998224 ) ) ;
#4203=ORIENTED_EDGE ( 'NONE', *, *, #4158, .T. ) ;
#4218=VERTEX_POINT ( 'NONE', #6139 ) ;
#4233=ORIENTED_EDGE ( 'NONE', *, *, #585, .T. ) ;
#4237=DIRECTION ( 'NONE',  ( 0.000000000000000000, 0.000000000000000000, 1.000000000000000000 ) ) ;
#4240=EDGE_CURVE ( 'NONE', #8931, #13447, #11644, .T. ) ;
#4255=DIRECTION ( 'NONE',  ( -0.000000000000000000, -0.000000000000000000, -1.000000000000000000 ) ) ;
#4288=CARTESIAN_POINT ( 'NONE',  ( -1.000000000000000000, -14.00000000000000000, 8.999999999999998224 ) ) ;
#4300=VERTEX_POINT ( 'NONE', #9505 ) ;
#4315=CIRCLE ( 'NONE', #4956, 1.499999999999999334 ) ;
#4323=DIRECTION ( 'NONE',  ( 1.000000000000000000, 0.000000000000000000, 0.000000000000000000 ) ) ;
#4329=EDGE_CURVE ( 'NONE', #1843, #11056, #310, .T. ) ;
#4334=FACE_OUTER_BOUND ( 'NONE', #7688, .T. ) ;
#4344=DIRECTION ( 'NONE',  ( -0.000000000000000000, -0.000000000000000000, -1.000000000000000000 ) ) ;
#4350=AXIS2_PLACEMENT_3D ( 'NONE', #6793, #9765, #1515 ) ;
#4351=DIRECTION ( 'NONE',  ( -1.000000000000000000, 0.000000000000000000, 0.000000000000000000 ) ) ;
#4364=ORIENTED_EDGE ( 'NONE', *, *, #6250, .T. ) ;
#4381=CARTESIAN_POINT ( 'NONE',  ( -7.500000000000013323, -7.009618943233427935, 9.000000000000000000 ) ) ;
#4413=EDGE_CURVE ( 'NONE', #7202, #9377, #3278, .T. ) ;
#4414=CARTESIAN_POINT ( 'NONE',  ( -8.759913291900476295, -7.823632761846195827, 9.000000000000000000 ) ) ;
#4419=AXIS2_PLACEMENT_3D ( 'NONE', #8502, #1074, #947 ) ;
#4428=DIRECTION ( 'NONE',  ( 0.000000000000000000, 0.000000000000000000, 1.000000000000000000 ) ) ;
#4432=ORIENTED_EDGE ( 'NONE', *, *, #13242, .F. ) ;
#4433=ORIENTED_EDGE ( 'NONE', *, *, #1650, .T. ) ;
#4467=AXIS2_PLACEMENT_3D ( 'NONE', #5849, #7984, #12196 ) ;
#4468=ORIENTED_EDGE ( 'NONE', *, *, #4827, .T. ) ;
#4470=VERTEX_POINT ( 'NONE', #3850 ) ;
#4474=( NAMED_UNIT ( * ) SI_UNIT ( $, .STERADIAN. ) SOLID_ANGLE_UNIT ( ) );
#4475=DIRECTION ( 'NONE',  ( 0.000000000000000000, 0.000000000000000000, 1.000000000000000000 ) ) ;
#4487=ORIENTED_EDGE ( 'NONE', *, *, #5916, .T. ) ;
#4488=DIRECTION ( 'NONE',  ( -0.000000000000000000, -0.000000000000000000, -1.000000000000000000 ) ) ;
#4497=ORIENTED_EDGE ( 'NONE', *, *, #10943, .T. ) ;
#4517=VECTOR ( 'NONE', #6446, 1000.000000000000000 ) ;
#4526=DIRECTION ( 'NONE',  ( -1.000000000000000000, 0.000000000000000000, 0.000000000000000000 ) ) ;
#4532=CARTESIAN_POINT ( 'NONE',  ( 6.165086708099361879, -6.325508935188243420, 0.000000000000000000 ) ) ;
#4550=DIRECTION ( 'NONE',  ( 0.000000000000000000, 0.000000000000000000, 1.000000000000000000 ) ) ;
#4555=VERTEX_POINT ( 'NONE', #6085 ) ;
#4559=DIRECTION ( 'NONE',  ( -9.858538378746663627E-23, 5.031452844637890958E-23, -1.000000000000000000 ) ) ;
#4560=CARTESIAN_POINT ( 'NONE',  ( -8.759913291900392807, -32.17636723815387256, 0.000000000000000000 ) ) ;
#4563=CARTESIAN_POINT ( 'NONE',  ( -12.99038105676654453, -27.50000000000006040, 9.000000000000000000 ) ) ;
#4591=ORIENTED_EDGE ( 'NONE', *, *, #9959, .T. ) ;
#4623=CIRCLE ( 'NONE', #848, 15.00000000000000000 ) ;
#4626=ORIENTED_EDGE ( 'NONE', *, *, #9234, .T. ) ;
#4627=ORIENTED_EDGE ( 'NONE', *, *, #9584, .T. ) ;
#4634=CARTESIAN_POINT ( 'NONE',  ( -7.499999999999923617, -32.99038105676662269, 9.000000000000000000 ) ) ;
#4657=VERTEX_POINT ( 'NONE', #13440 ) ;
#4659=VERTEX_POINT ( 'NONE', #998 ) ;
#4668=CARTESIAN_POINT ( 'NONE',  ( -12.99038105676659427, -12.50000000000003020, -9.000000000000000000 ) ) ;
#4679=ADVANCED_FACE ( 'NONE', ( #10415, #7451 ), #11655, .F. ) ;
#4681=CYLINDRICAL_SURFACE ( 'NONE', #10187, 1.500000000000001332 ) ;
#4688=CARTESIAN_POINT ( 'NONE',  ( 14.92499999999998650, -18.50187617334198009, 0.000000000000000000 ) ) ;
#4718=DIRECTION ( 'NONE',  ( -0.000000000000000000, -0.000000000000000000, 1.000000000000000000 ) ) ;
#4719=DIRECTION ( 'NONE',  ( -4.082155997157844188E-16, 1.000000000000000000, 0.000000000000000000 ) ) ;
#4724=FACE_OUTER_BOUND ( 'NONE', #8254, .T. ) ;
#4738=CARTESIAN_POINT ( 'NONE',  ( 2.449293598294706513E-15, -5.000000000000000888, -9.000000000000000000 ) ) ;
#4744=AXIS2_PLACEMENT_3D ( 'NONE', #9654, #1262, #5513 ) ;
#4756=DIRECTION ( 'NONE',  ( 1.000000000000000000, 0.000000000000000000, 0.000000000000000000 ) ) ;
#4761=EDGE_CURVE ( 'NONE', #1857, #2588, #3862, .T. ) ;
#4763=ORIENTED_EDGE ( 'NONE', *, *, #11996, .F. ) ;
#4777=ORIENTED_EDGE ( 'NONE', *, *, #5591, .T. ) ;
#4783=CARTESIAN_POINT ( 'NONE',  ( 12.17636723815389566, -28.75991329190035373, 0.000000000000000000 ) ) ;
#4791=EDGE_CURVE ( 'NONE', #11878, #11056, #5359, .T. ) ;
#4795=ORIENTED_EDGE ( 'NONE', *, *, #11342, .T. ) ;
#4805=CARTESIAN_POINT ( 'NONE',  ( 2.449293598294706513E-15, -20.00000000000000000, 15.00000000000000355 ) ) ;
#4813=EDGE_LOOP ( 'NONE', ( #5808, #796, #4468, #11877 ) ) ;
#4817=CARTESIAN_POINT ( 'NONE',  ( -13.67449106481164733, -26.16508670809959725, 9.000000000000000000 ) ) ;
#4821=DIRECTION ( 'NONE',  ( 0.000000000000000000, 0.000000000000000000, -1.000000000000000000 ) ) ;
#4827=EDGE_CURVE ( 'NONE', #10268, #582, #9540, .T. ) ;
#4830=CARTESIAN_POINT ( 'NONE',  ( 14.92499999999998650, -18.50187617334196943, -9.000000000000000000 ) ) ;
#4833=CARTESIAN_POINT ( 'NONE',  ( 5.000000000000003553, -20.00000000000000000, 15.00000000000000355 ) ) ;
#4853=CARTESIAN_POINT ( 'NONE',  ( -5.999999999999921840, -32.99038105676662269, -9.000000000000000000 ) ) ;
#4857=CIRCLE ( 'NONE', #8393, 1.499999999999999334 ) ;
#4866=ORIENTED_EDGE ( 'NONE', *, *, #7550, .T. ) ;
#4872=CARTESIAN_POINT ( 'NONE',  ( -1.000000000000000000, -14.00000000000000000, -9.000000000000001776 ) ) ;
#4879=DIRECTION ( 'NONE',  ( 0.8660254037844450359, -0.4999999999999888423, 0.000000000000000000 ) ) ;
#4890=DIRECTION ( 'NONE',  ( -0.8660254037844355990, -0.5000000000000055511, 0.000000000000000000 ) ) ;
#4904=CYLINDRICAL_SURFACE ( 'NONE', #6816, 1.500000000000000444 ) ;
#4907=AXIS2_PLACEMENT_3D ( 'NONE', #2649, #6871, #11079 ) ;
#4956=AXIS2_PLACEMENT_3D ( 'NONE', #3643, #5794, #6693 ) ;
#4959=VERTEX_POINT ( 'NONE', #3004 ) ;
#4986=CIRCLE ( 'NONE', #13102, 15.00000000000000000 ) ;
#4996=CARTESIAN_POINT ( 'NONE',  ( -5.999999999999921840, -32.99038105676662269, 9.000000000000000000 ) ) ;
#5006=ORIENTED_EDGE ( 'NONE', *, *, #9483, .T. ) ;
#5009=UNCERTAINTY_MEASURE_WITH_UNIT (LENGTH_MEASURE( 1.000000000000000082E-05 ), #9177, 'distance_accuracy_value', 'NONE');
#5014=EDGE_CURVE ( 'NONE', #2384, #4657, #921, .T. ) ;
#5015=CARTESIAN_POINT ( 'NONE',  ( -12.99038105676654453, -27.50000000000006040, 9.000000000000000000 ) ) ;
#5037=DIRECTION ( 'NONE',  ( -0.000000000000000000, -0.000000000000000000, -1.000000000000000000 ) ) ;
#5039=DIRECTION ( 'NONE',  ( 1.000000000000000000, 0.000000000000000000, 0.000000000000000000 ) ) ;
#5075=VECTOR ( 'NONE', #5634, 1000.000000000000000 ) ;
#5076=ORIENTED_EDGE ( 'NONE', *, *, #9792, .F. ) ;
#5084=DIRECTION ( 'NONE',  ( 0.000000000000000000, 0.000000000000000000, 1.000000000000000000 ) ) ;
#5090=CARTESIAN_POINT ( 'NONE',  ( -14.92500000000000249, -18.50187617334218970, 0.000000000000000000 ) ) ;
#5099=ORIENTED_EDGE ( 'NONE', *, *, #4240, .F. ) ;
#5107=DIRECTION ( 'NONE',  ( 1.000000000000000000, 0.000000000000000000, 0.000000000000000000 ) ) ;
#5138=CARTESIAN_POINT ( 'NONE',  ( -7.499999999999923617, -32.99038105676662269, -9.000000000000000000 ) ) ;
#5171=CARTESIAN_POINT ( 'NONE',  ( -1.498123826657872470, -5.075000000000001066, -9.000000000000000000 ) ) ;
#5198=CYLINDRICAL_SURFACE ( 'NONE', #13662, 1.500000000000001332 ) ;
#5207=VERTEX_POINT ( 'NONE', #415 ) ;
#5232=CARTESIAN_POINT ( 'NONE',  ( -14.99999999999999645, -20.00000000000005329, -9.000000000000000000 ) ) ;
#5245=VECTOR ( 'NONE', #3743, 1000.000000000000000 ) ;
#5253=VERTEX_POINT ( 'NONE', #11837 ) ;
#5267=ADVANCED_FACE ( 'NONE', ( #7839 ), #1312, .T. ) ;
#5269=ADVANCED_FACE ( 'NONE', ( #4724 ), #9837, .F. ) ;
#5280=VECTOR ( 'NONE', #8206, 1000.000000000000000 ) ;
#5294=CIRCLE ( 'NONE', #3297, 1.500000000000001110 ) ;
#5297=CARTESIAN_POINT ( 'NONE',  ( 14.92499999999998650, -18.50187617334198009, 9.000000000000000000 ) ) ;
#5306=CARTESIAN_POINT ( 'NONE',  ( -12.99038105676654453, -27.50000000000006040, -9.000000000000000000 ) ) ;
#5317=ORIENTED_EDGE ( 'NONE', *, *, #9234, .F. ) ;
#5320=VECTOR ( 'NONE', #4756, 1000.000000000000000 ) ;
#5321=FACE_OUTER_BOUND ( 'NONE', #1879, .T. ) ;
#5326=EDGE_CURVE ( 'NONE', #7674, #7202, #7109, .T. ) ;
#5352=FACE_OUTER_BOUND ( 'NONE', #552, .T. ) ;
#5359=CIRCLE ( 'NONE', #8882, 15.00000000000000000 ) ;
#5391=CLOSED_SHELL ( 'NONE', ( #2239, #2401, #9796, #7868, #2600, #6860, #10966, #8008, #7639, #1097, #5267, #10324, #1095, #11114, #19, #10060, #297, #8036, #9928, #5532, #4679, #12368, #10672, #7299, #9542, #5439, #10422, #8088, #7691, #8897, #12890, #6773, #120, #2736, #3794, #5269, #2605 ) ) ;
#5394=DIRECTION ( 'NONE',  ( 0.000000000000000000, 0.000000000000000000, -1.000000000000000000 ) ) ;
#5404=AXIS2_PLACEMENT_3D ( 'NONE', #5306, #6415, #4323 ) ;
#5409=LINE ( 'NONE', #2202, #4517 ) ;
#5412=AXIS2_PLACEMENT_3D ( 'NONE', #10944, #7709, #2438 ) ;
#5415=AXIS2_PLACEMENT_3D ( 'NONE', #6410, #12673, #8201 ) ;
#5422=AXIS2_PLACEMENT_3D ( 'NONE', #4071, #11465, #13658 ) ;
#5428=FACE_BOUND ( 'NONE', #1247, .T. ) ;
#5431=DIRECTION ( 'NONE',  ( -0.000000000000000000, 0.000000000000000000, -1.000000000000000000 ) ) ;
#5439=ADVANCED_FACE ( 'NONE', ( #5976 ), #7904, .F. ) ;
#5469=ORIENTED_EDGE ( 'NONE', *, *, #6407, .T. ) ;
#5472=DIRECTION ( 'NONE',  ( 0.000000000000000000, 0.000000000000000000, 1.000000000000000000 ) ) ;
#5504=DIRECTION ( 'NONE',  ( 0.000000000000000000, 0.000000000000000000, 1.000000000000000000 ) ) ;
#5510=FACE_OUTER_BOUND ( 'NONE', #10923, .T. ) ;
#5513=DIRECTION ( 'NONE',  ( 1.000000000000000000, 0.000000000000000000, 0.000000000000000000 ) ) ;
#5514=ORIENTED_EDGE ( 'NONE', *, *, #2577, .T. ) ;
#5518=CARTESIAN_POINT ( 'NONE',  ( -8.759913291900476295, -7.823632761846195827, 0.000000000000000000 ) ) ;
#5521=CARTESIAN_POINT ( 'NONE',  ( -12.17636723815377309, -28.75991329190052070, 9.000000000000000000 ) ) ;
#5532=ADVANCED_FACE ( 'NONE', ( #11139 ), #193, .T. ) ;
#5533=ORIENTED_EDGE ( 'NONE', *, *, #7633, .T. ) ;
#5536=CARTESIAN_POINT ( 'NONE',  ( -13.67449106481164733, -26.16508670809959725, 0.000000000000000000 ) ) ;
#5564=CARTESIAN_POINT ( 'NONE',  ( 1.498123826657866253, -34.92499999999999716, 0.000000000000000000 ) ) ;
#5574=DIRECTION ( 'NONE',  ( -0.8660254037844355990, -0.5000000000000055511, 0.000000000000000000 ) ) ;
#5582=ORIENTED_EDGE ( 'NONE', *, *, #6250, .F. ) ;
#5586=CARTESIAN_POINT ( 'NONE',  ( -0.9999999999999995559, -15.10102051443364246, 9.000000000000000000 ) ) ;
#5587=CARTESIAN_POINT ( 'NONE',  ( 7.499999999999834799, -7.009618943233325794, -9.000000000000000000 ) ) ;
#5588=SURFACE_STYLE_USAGE ( .BOTH. , #10761 ) ;
#5589=CARTESIAN_POINT ( 'NONE',  ( -14.99999999999999645, -20.00000000000005329, -9.000000000000000000 ) ) ;
#5591=EDGE_CURVE ( 'NONE', #11391, #5893, #8655, .T. ) ;
#5604=CARTESIAN_POINT ( 'NONE',  ( 2.449293598294706513E-15, -20.00000000000000000, 9.000000000000000000 ) ) ;
#5628=CARTESIAN_POINT ( 'NONE',  ( -0.9999999999999976685, -20.00000000000000000, 8.999999999999998224 ) ) ;
#5629=CARTESIAN_POINT ( 'NONE',  ( 2.449293598294706513E-15, -20.00000000000000000, -9.000000000000000000 ) ) ;
#5634=DIRECTION ( 'NONE',  ( -0.000000000000000000, -0.000000000000000000, 1.000000000000000000 ) ) ;
#5635=AXIS2_PLACEMENT_3D ( 'NONE', #1061, #13585, #5039 ) ;
#5654=ORIENTED_EDGE ( 'NONE', *, *, #1220, .T. ) ;
#5655=LINE ( 'NONE', #11307, #5280 ) ;
#5668=ORIENTED_EDGE ( 'NONE', *, *, #11597, .T. ) ;
#5690=CARTESIAN_POINT ( 'NONE',  ( 6.165086708099361879, -6.325508935188243420, 9.000000000000000000 ) ) ;
#5706=CARTESIAN_POINT ( 'NONE',  ( 1.000000000000002442, -20.00000000000000000, 8.999999999999998224 ) ) ;
#5717=CARTESIAN_POINT ( 'NONE',  ( -11.49038105676659249, -12.50000000000003020, -9.000000000000000000 ) ) ;
#5747=CIRCLE ( 'NONE', #4419, 1.500000000000000666 ) ;
#5753=ORIENTED_EDGE ( 'NONE', *, *, #2913, .F. ) ;
#5754=ORIENTED_EDGE ( 'NONE', *, *, #846, .F. ) ;
#5755=ORIENTED_EDGE ( 'NONE', *, *, #3985, .F. ) ;
#5778=VECTOR ( 'NONE', #6965, 1000.000000000000000 ) ;
#5790=AXIS2_PLACEMENT_3D ( 'NONE', #2428, #13073, #483 ) ;
#5792=ORIENTED_EDGE ( 'NONE', *, *, #8609, .F. ) ;
#5793=CYLINDRICAL_SURFACE ( 'NONE', #12977, 1.500000000000000444 ) ;
#5794=DIRECTION ( 'NONE',  ( 0.000000000000000000, 0.000000000000000000, 1.000000000000000000 ) ) ;
#5808=ORIENTED_EDGE ( 'NONE', *, *, #13277, .F. ) ;
#5813=CARTESIAN_POINT ( 'NONE',  ( -7.499999999999923617, -32.99038105676662269, -9.000000000000000000 ) ) ;
#5827=FACE_OUTER_BOUND ( 'NONE', #7940, .T. ) ;
#5828=CARTESIAN_POINT ( 'NONE',  ( 0.000000000000000000, 0.000000000000000000, 0.000000000000000000 ) ) ;
#5831=CARTESIAN_POINT ( 'NONE',  ( -8.759913291900394583, -32.17636723815387256, -9.000000000000000000 ) ) ;
#5841=ORIENTED_EDGE ( 'NONE', *, *, #10069, .T. ) ;
#5844=DIRECTION ( 'NONE',  ( -9.858538378746663627E-23, 5.031452844637890958E-23, -1.000000000000000000 ) ) ;
#5849=CARTESIAN_POINT ( 'NONE',  ( 2.449293598294706513E-15, -5.000000000000000888, 9.000000000000000000 ) ) ;
#5851=CIRCLE ( 'NONE', #5412, 15.00000000000000000 ) ;
#5853=DIRECTION ( 'NONE',  ( 0.000000000000000000, 0.000000000000000000, 1.000000000000000000 ) ) ;
#5857=EDGE_CURVE ( 'NONE', #13447, #6557, #3943, .T. ) ;
#5879=DIRECTION ( 'NONE',  ( 0.000000000000000000, -0.000000000000000000, 1.000000000000000000 ) ) ;
#5893=VERTEX_POINT ( 'NONE', #8282 ) ;
#5909=CARTESIAN_POINT ( 'NONE',  ( 12.17636723815370736, -11.24008670809938693, -9.000000000000000000 ) ) ;
#5916=EDGE_CURVE ( 'NONE', #6266, #5253, #3287, .T. ) ;
#5917=DIRECTION ( 'NONE',  ( 0.000000000000000000, 0.000000000000000000, 1.000000000000000000 ) ) ;
#5922=ORIENTED_EDGE ( 'NONE', *, *, #3394, .T. ) ;
#5924=ORIENTED_EDGE ( 'NONE', *, *, #8072, .T. ) ;
#5933=DIRECTION ( 'NONE',  ( -0.000000000000000000, 0.000000000000000000, -1.000000000000000000 ) ) ;
#5944=ORIENTED_EDGE ( 'NONE', *, *, #13033, .F. ) ;
#5948=AXIS2_PLACEMENT_3D ( 'NONE', #8746, #8101, #1648 ) ;
#5956=EDGE_CURVE ( 'NONE', #439, #10938, #9254, .T. ) ;
#5961=ORIENTED_EDGE ( 'NONE', *, *, #2646, .T. ) ;
#5962=ORIENTED_EDGE ( 'NONE', *, *, #7591, .F. ) ;
#5968=DIRECTION ( 'NONE',  ( 0.000000000000000000, 0.000000000000000000, 1.000000000000000000 ) ) ;
#5975=STYLED_ITEM('',(#13691),#961);
#5976=FACE_OUTER_BOUND ( 'NONE', #3535, .T. ) ;
#5984=DIRECTION ( 'NONE',  ( 0.000000000000000000, 0.000000000000000000, 1.000000000000000000 ) ) ;
#5991=CARTESIAN_POINT ( 'NONE',  ( 2.449293598294706513E-15, -20.00000000000000000, 9.000000000000000000 ) ) ;
#6010=AXIS2_PLACEMENT_3D ( 'NONE', #11238, #1758, #10275 ) ;
#6016=CARTESIAN_POINT ( 'NONE',  ( -7.500000000000013323, -7.009618943233427935, -9.000000000000000000 ) ) ;
#6023=AXIS2_PLACEMENT_3D ( 'NONE', #8942, #11982, #8800 ) ;
#6031=EDGE_CURVE ( 'NONE', #3891, #6039, #5294, .T. ) ;
#6039=VERTEX_POINT ( 'NONE', #11923 ) ;
#6042=DIRECTION ( 'NONE',  ( 0.000000000000000000, 0.000000000000000000, -1.000000000000000000 ) ) ;
#6060=CARTESIAN_POINT ( 'NONE',  ( 2.449293598294706513E-15, -35.00000000000000000, -9.000000000000000000 ) ) ;
#6069=CARTESIAN_POINT ( 'NONE',  ( 2.449293598294706513E-15, -20.00000000000000000, 9.000000000000000000 ) ) ;
#6082=AXIS2_PLACEMENT_3D ( 'NONE', #2149, #8526, #9491 ) ;
#6085=CARTESIAN_POINT ( 'NONE',  ( 14.92500000000001492, -21.49812382665770727, 9.000000000000000000 ) ) ;
#6089=VECTOR ( 'NONE', #1992, 1000.000000000000000 ) ;
#6092=AXIS2_PLACEMENT_3D ( 'NONE', #265, #5472, #9675 ) ;
#6117=DIRECTION ( 'NONE',  ( 0.8660254037844381525, 0.5000000000000009992, 0.000000000000000000 ) ) ;
#6119=AXIS2_PLACEMENT_3D ( 'NONE', #5991, #3632, #625 ) ;
#6124=ORIENTED_EDGE ( 'NONE', *, *, #1650, .F. ) ;
#6139=CARTESIAN_POINT ( 'NONE',  ( 8.759913291900311094, -7.823632761846075923, -9.000000000000000000 ) ) ;
#6173=VECTOR ( 'NONE', #1474, 1000.000000000000000 ) ;
#6179=FACE_OUTER_BOUND ( 'NONE', #1881, .T. ) ;
#6196=DIRECTION ( 'NONE',  ( -1.000000000000000000, 0.000000000000000000, 0.000000000000000000 ) ) ;
#6203=DIRECTION ( 'NONE',  ( -0.000000000000000000, -0.000000000000000000, -1.000000000000000000 ) ) ;
#6250=EDGE_CURVE ( 'NONE', #10723, #4470, #4623, .T. ) ;
#6252=AXIS2_PLACEMENT_3D ( 'NONE', #12948, #2443, #11788 ) ;
#6256=CARTESIAN_POINT ( 'NONE',  ( 1.000000000000000444, -15.10102051443364246, 9.000000000000000000 ) ) ;
#6266=VERTEX_POINT ( 'NONE', #8126 ) ;
#6287=CARTESIAN_POINT ( 'NONE',  ( -12.17636723815382993, -11.24008670809956456, 0.000000000000000000 ) ) ;
#6294=CARTESIAN_POINT ( 'NONE',  ( 2.449293598294706513E-15, -20.00000000000000000, -9.000000000000000000 ) ) ;
#6300=DIRECTION ( 'NONE',  ( -0.000000000000000000, -0.000000000000000000, 1.000000000000000000 ) ) ;
#6305=CIRCLE ( 'NONE', #11588, 15.00000000000000000 ) ;
#6312=CIRCLE ( 'NONE', #5422, 1.499999999999999778 ) ;
#6315=AXIS2_PLACEMENT_3D ( 'NONE', #6294, #9449, #2175 ) ;
#6336=CARTESIAN_POINT ( 'NONE',  ( -12.17636723815377309, -28.75991329190052070, 0.000000000000000000 ) ) ;
#6348=CARTESIAN_POINT ( 'NONE',  ( 2.449293598294706513E-15, -20.00000000000000000, 9.000000000000000000 ) ) ;
#6351=CARTESIAN_POINT ( 'NONE',  ( -6.165086708099452473, -33.67449106481171128, 0.000000000000000000 ) ) ;
#6356=DIRECTION ( 'NONE',  ( 0.000000000000000000, 0.000000000000000000, 1.000000000000000000 ) ) ;
#6392=VERTEX_POINT ( 'NONE', #5297 ) ;
#6394=DIRECTION ( 'NONE',  ( -0.000000000000000000, -0.000000000000000000, -1.000000000000000000 ) ) ;
#6397=DIRECTION ( 'NONE',  ( -1.000000000000000000, 0.000000000000000000, 0.000000000000000000 ) ) ;
#6398=DIRECTION ( 'NONE',  ( -0.000000000000000000, -0.000000000000000000, -1.000000000000000000 ) ) ;
#6407=EDGE_CURVE ( 'NONE', #5893, #2278, #4044, .T. ) ;
#6410=CARTESIAN_POINT ( 'NONE',  ( 12.99038105676665289, -27.49999999999988276, -9.000000000000000000 ) ) ;
#6415=DIRECTION ( 'NONE',  ( 0.000000000000000000, -0.000000000000000000, 1.000000000000000000 ) ) ;
#6446=DIRECTION ( 'NONE',  ( -0.000000000000000000, -0.000000000000000000, 1.000000000000000000 ) ) ;
#6455=AXIS2_PLACEMENT_3D ( 'NONE', #6661, #10991, #1513 ) ;
#6458=ORIENTED_EDGE ( 'NONE', *, *, #5956, .T. ) ;
#6478=VERTEX_POINT ( 'NONE', #4996 ) ;
#6481=DIRECTION ( 'NONE',  ( -0.000000000000000000, 0.000000000000000000, -1.000000000000000000 ) ) ;
#6485=FACE_OUTER_BOUND ( 'NONE', #11128, .T. ) ;
#6494=VERTEX_POINT ( 'NONE', #812 ) ;
#6496=ORIENTED_EDGE ( 'NONE', *, *, #4413, .F. ) ;
#6517=CIRCLE ( 'NONE', #8283, 1.499999999999999334 ) ;
#6544=EDGE_CURVE ( 'NONE', #2116, #13409, #6925, .T. ) ;
#6549=CYLINDRICAL_SURFACE ( 'NONE', #10607, 15.00000000000000000 ) ;
#6551=CARTESIAN_POINT ( 'NONE',  ( -6.000000000000012434, -7.009618943233427935, 9.000000000000000000 ) ) ;
#6556=AXIS2_PLACEMENT_3D ( 'NONE', #4805, #8125, #1466 ) ;
#6557=VERTEX_POINT ( 'NONE', #12243 ) ;
#6566=CARTESIAN_POINT ( 'NONE',  ( -14.99999999999999645, -20.00000000000005329, 9.000000000000000000 ) ) ;
#6571=VERTEX_POINT ( 'NONE', #1867 ) ;
#6580=DIRECTION ( 'NONE',  ( 0.000000000000000000, 0.000000000000000000, 1.000000000000000000 ) ) ;
#6585=VECTOR ( 'NONE', #3100, 1000.000000000000000 ) ;
#6591=CARTESIAN_POINT ( 'NONE',  ( 14.92500000000001492, -21.49812382665770727, 0.000000000000000000 ) ) ;
#6599=VERTEX_POINT ( 'NONE', #4853 ) ;
#6602=ORIENTED_EDGE ( 'NONE', *, *, #9608, .F. ) ;
#6633=VECTOR ( 'NONE', #7908, 1000.000000000000000 ) ;
#6642=ORIENTED_EDGE ( 'NONE', *, *, #769, .F. ) ;
#6643=ORIENTED_EDGE ( 'NONE', *, *, #7030, .F. ) ;
#6661=CARTESIAN_POINT ( 'NONE',  ( 7.500000000000107470, -32.99038105676652322, -9.000000000000000000 ) ) ;
#6666=DIRECTION ( 'NONE',  ( 4.082155997157843695E-16, -1.000000000000000000, 0.000000000000000000 ) ) ;
#6674=AXIS2_PLACEMENT_3D ( 'NONE', #5628, #10794, #6666 ) ;
#6675=DIRECTION ( 'NONE',  ( 0.000000000000000000, 0.000000000000000000, 1.000000000000000000 ) ) ;
#6693=DIRECTION ( 'NONE',  ( -0.5000000000000041078, 0.8660254037844362651, 0.000000000000000000 ) ) ;
#6711=DIRECTION ( 'NONE',  ( 0.000000000000000000, -0.000000000000000000, 1.000000000000000000 ) ) ;
#6714=DIRECTION ( 'NONE',  ( -0.5000000000000041078, 0.8660254037844362651, 0.000000000000000000 ) ) ;
#6722=ORIENTED_EDGE ( 'NONE', *, *, #11342, .F. ) ;
#6726=CIRCLE ( 'NONE', #2741, 15.00000000000000000 ) ;
#6737=ORIENTED_EDGE ( 'NONE', *, *, #7704, .F. ) ;
#6738=CARTESIAN_POINT ( 'NONE',  ( -1.498123826657861368, -34.92499999999999716, 0.000000000000000000 ) ) ;
#6771=ORIENTED_EDGE ( 'NONE', *, *, #4791, .F. ) ;
#6773=ADVANCED_FACE ( 'NONE', ( #2006 ), #7276, .F. ) ;
#6783=ORIENTED_EDGE ( 'NONE', *, *, #4008, .F. ) ;
#6793=CARTESIAN_POINT ( 'NONE',  ( 2.449293598294706513E-15, -20.00000000000000000, 9.000000000000000000 ) ) ;
#6810=DIRECTION ( 'NONE',  ( 1.000000000000000000, 0.000000000000000000, 0.000000000000000000 ) ) ;
#6811=CARTESIAN_POINT ( 'NONE',  ( 2.449293598294706513E-15, -20.00000000000000000, 9.000000000000000000 ) ) ;
#6816=AXIS2_PLACEMENT_3D ( 'NONE', #6016, #6300, #12495 ) ;
#6818=CARTESIAN_POINT ( 'NONE',  ( -6.165086708099547508, -6.325508935188330462, -9.000000000000000000 ) ) ;
#6835=AXIS2_PLACEMENT_3D ( 'NONE', #5813, #5879, #3720 ) ;
#6846=EDGE_CURVE ( 'NONE', #13409, #10472, #7561, .T. ) ;
#6848=EDGE_LOOP ( 'NONE', ( #8326, #7827, #10216, #4626 ) ) ;
#6860=ADVANCED_FACE ( 'NONE', ( #6179 ), #887, .F. ) ;
#6863=DIRECTION ( 'NONE',  ( -0.000000000000000000, -0.000000000000000000, 1.000000000000000000 ) ) ;
#6870=DIRECTION ( 'NONE',  ( -1.000000000000000000, 0.000000000000000000, 0.000000000000000000 ) ) ;
#6871=DIRECTION ( 'NONE',  ( 0.000000000000000000, 0.000000000000000000, 1.000000000000000000 ) ) ;
#6881=DIRECTION ( 'NONE',  ( 0.000000000000000000, 0.000000000000000000, 1.000000000000000000 ) ) ;
#6883=CIRCLE ( 'NONE', #13046, 5.000000000000000888 ) ;
#6896=VECTOR ( 'NONE', #25, 1000.000000000000000 ) ;
#6925=LINE ( 'NONE', #9069, #2918 ) ;
#6927=CARTESIAN_POINT ( 'NONE',  ( 13.67449106481173615, -26.16508670809940895, 9.000000000000000000 ) ) ;
#6939=EDGE_LOOP ( 'NONE', ( #3028, #3733, #3368, #198 ) ) ;
#6947=EDGE_CURVE ( 'NONE', #6494, #12390, #8895, .T. ) ;
#6965=DIRECTION ( 'NONE',  ( -0.000000000000000000, -0.000000000000000000, 1.000000000000000000 ) ) ;
#6979=DIRECTION ( 'NONE',  ( -0.000000000000000000, -0.000000000000000000, -1.000000000000000000 ) ) ;
#6985=DIRECTION ( 'NONE',  ( -1.000000000000000000, -4.082155997157843695E-16, 0.000000000000000000 ) ) ;
#6987=VERTEX_POINT ( 'NONE', #4817 ) ;
#6988=ORIENTED_EDGE ( 'NONE', *, *, #689, .T. ) ;
#6990=EDGE_LOOP ( 'NONE', ( #9553, #8439, #8556, #1680 ) ) ;
#7008=ORIENTED_EDGE ( 'NONE', *, *, #9951, .T. ) ;
#7009=CARTESIAN_POINT ( 'NONE',  ( 2.449293598294706513E-15, -20.00000000000000000, 9.000000000000000000 ) ) ;
#7010=DIRECTION ( 'NONE',  ( 1.000000000000000000, 0.000000000000000000, 0.000000000000000000 ) ) ;
#7013=CARTESIAN_POINT ( 'NONE',  ( 7.499999999999834799, -7.009618943233325794, 9.000000000000000000 ) ) ;
#7015=DIRECTION ( 'NONE',  ( 1.000000000000000000, 0.000000000000000000, 0.000000000000000000 ) ) ;
#7030=EDGE_CURVE ( 'NONE', #6571, #4657, #3577, .T. ) ;
#7031=CARTESIAN_POINT ( 'NONE',  ( -14.92499999999998828, -21.49812382665791688, 0.000000000000000000 ) ) ;
#7075=ORIENTED_EDGE ( 'NONE', *, *, #12859, .F. ) ;
#7076=VECTOR ( 'NONE', #929, 1000.000000000000000 ) ;
#7079=VERTEX_POINT ( 'NONE', #9528 ) ;
#7081=DIRECTION ( 'NONE',  ( 0.000000000000000000, 0.000000000000000000, 1.000000000000000000 ) ) ;
#7088=DIRECTION ( 'NONE',  ( 0.000000000000000000, 0.000000000000000000, 1.000000000000000000 ) ) ;
#7093=ORIENTED_EDGE ( 'NONE', *, *, #9827, .T. ) ;
#7109=CIRCLE ( 'NONE', #6023, 1.500000000000001332 ) ;
#7113=CARTESIAN_POINT ( 'NONE',  ( -13.67449106481168997, -13.83491329190049690, 9.000000000000000000 ) ) ;
#7136=EDGE_CURVE ( 'NONE', #1508, #278, #7596, .T. ) ;
#7153=CARTESIAN_POINT ( 'NONE',  ( 2.449293598294706513E-15, -20.00000000000000000, 9.000000000000000000 ) ) ;
#7167=VERTEX_POINT ( 'NONE', #7662 ) ;
#7171=DIRECTION ( 'NONE',  ( -1.000000000000000000, 0.000000000000000000, 0.000000000000000000 ) ) ;
#7177=AXIS2_PLACEMENT_3D ( 'NONE', #7009, #11426, #13486 ) ;
#7192=EDGE_LOOP ( 'NONE', ( #2522, #5469, #13654, #5792 ) ) ;
#7200=DIRECTION ( 'NONE',  ( 0.000000000000000000, 0.000000000000000000, 1.000000000000000000 ) ) ;
#7202=VERTEX_POINT ( 'NONE', #13228 ) ;
#7223=DIRECTION ( 'NONE',  ( -1.000000000000000000, 0.000000000000000000, 0.000000000000000000 ) ) ;
#7225=CARTESIAN_POINT ( 'NONE',  ( -11.49038105676659249, -12.50000000000003020, 9.000000000000000000 ) ) ;
#7243=CYLINDRICAL_SURFACE ( 'NONE', #9470, 15.00000000000000000 ) ;
#7254=AXIS2_PLACEMENT_3D ( 'NONE', #2773, #2627, #476 ) ;
#7260=CARTESIAN_POINT ( 'NONE',  ( -4.999999999999998224, -20.00000000000000000, 9.000000000000000000 ) ) ;
#7276=CYLINDRICAL_SURFACE ( 'NONE', #3148, 1.500000000000001332 ) ;
#7295=VECTOR ( 'NONE', #5431, 1000.000000000000000 ) ;
#7299=ADVANCED_FACE ( 'NONE', ( #9862 ), #4681, .F. ) ;
#7311=ORIENTED_EDGE ( 'NONE', *, *, #2913, .T. ) ;
#7321=VECTOR ( 'NONE', #10976, 1000.000000000000000 ) ;
#7324=DIRECTION ( 'NONE',  ( 1.000000000000000000, 0.000000000000000000, 0.000000000000000000 ) ) ;
#7342=CIRCLE ( 'NONE', #10850, 1.500000000000001332 ) ;
#7402=CARTESIAN_POINT ( 'NONE',  ( 12.99038105676649835, -12.49999999999984901, -9.000000000000000000 ) ) ;
#7403=CIRCLE ( 'NONE', #965, 15.00000000000000000 ) ;
#7444=CYLINDRICAL_SURFACE ( 'NONE', #5404, 1.500000000000001332 ) ;
#7450=EDGE_CURVE ( 'NONE', #8931, #12388, #453, .T. ) ;
#7451=FACE_OUTER_BOUND ( 'NONE', #13322, .T. ) ;
#7467=DIRECTION ( 'NONE',  ( -0.000000000000000000, -0.000000000000000000, 1.000000000000000000 ) ) ;
#7469=CARTESIAN_POINT ( 'NONE',  ( -7.500000000000013323, -7.009618943233427935, -9.000000000000000000 ) ) ;
#7474=AXIS2_PLACEMENT_3D ( 'NONE', #11199, #672, #1510 ) ;
#7483=ORIENTED_EDGE ( 'NONE', *, *, #2362, .T. ) ;
#7484=AXIS2_PLACEMENT_3D ( 'NONE', #927, #13437, #1975 ) ;
#7498=CARTESIAN_POINT ( 'NONE',  ( -11.49038105676654453, -27.50000000000006040, 9.000000000000000000 ) ) ;
#7524=CIRCLE ( 'NONE', #9067, 1.500000000000000666 ) ;
#7526=DIRECTION ( 'NONE',  ( -3.469446951953611033E-15, 1.000000000000000000, 0.000000000000000000 ) ) ;
#7527=CARTESIAN_POINT ( 'NONE',  ( 1.000000000000000444, -15.10102051443364246, 15.00000000000000355 ) ) ;
#7540=LINE ( 'NONE', #335, #231 ) ;
#7550=EDGE_CURVE ( 'NONE', #13409, #4218, #11055, .T. ) ;
#7558=CARTESIAN_POINT ( 'NONE',  ( 2.449293598294706513E-15, -20.00000000000000000, -9.000000000000000000 ) ) ;
#7561=CIRCLE ( 'NONE', #11075, 1.500000000000001554 ) ;
#7571=ORIENTED_EDGE ( 'NONE', *, *, #12859, .T. ) ;
#7586=AXIS2_PLACEMENT_3D ( 'NONE', #12300, #7200, #10157 ) ;
#7588=ORIENTED_EDGE ( 'NONE', *, *, #9499, .F. ) ;
#7591=EDGE_CURVE ( 'NONE', #10020, #12390, #3555, .T. ) ;
#7596=LINE ( 'NONE', #7527, #895 ) ;
#7621=ORIENTED_EDGE ( 'NONE', *, *, #9499, .T. ) ;
#7627=CYLINDRICAL_SURFACE ( 'NONE', #4350, 15.00000000000000000 ) ;
#7633=EDGE_CURVE ( 'NONE', #10628, #10472, #13039, .T. ) ;
#7639=ADVANCED_FACE ( 'NONE', ( #3422 ), #7710, .T. ) ;
#7644=CARTESIAN_POINT ( 'NONE',  ( 2.449293598294706513E-15, -20.00000000000000000, 9.000000000000000000 ) ) ;
#7649=CARTESIAN_POINT ( 'NONE',  ( 7.500000000000107470, -32.99038105676652322, -9.000000000000000000 ) ) ;
#7661=DIRECTION ( 'NONE',  ( -0.000000000000000000, -0.000000000000000000, 1.000000000000000000 ) ) ;
#7662=CARTESIAN_POINT ( 'NONE',  ( 5.000000000000003553, -20.00000000000000000, -8.999999999999998224 ) ) ;
#7663=CARTESIAN_POINT ( 'NONE',  ( 12.99038105676649835, -12.49999999999984901, -9.000000000000000000 ) ) ;
#7672=ORIENTED_EDGE ( 'NONE', *, *, #4761, .T. ) ;
#7673=VERTEX_POINT ( 'NONE', #1813 ) ;
#7674=VERTEX_POINT ( 'NONE', #694 ) ;
#7688=EDGE_LOOP ( 'NONE', ( #881, #7995, #12737, #9219 ) ) ;
#7691=ADVANCED_FACE ( 'NONE', ( #13417 ), #13285, .F. ) ;
#7704=EDGE_CURVE ( 'NONE', #10628, #2996, #7342, .T. ) ;
#7706=DIRECTION ( 'NONE',  ( -0.000000000000000000, -0.000000000000000000, 1.000000000000000000 ) ) ;
#7709=DIRECTION ( 'NONE',  ( 0.000000000000000000, 0.000000000000000000, 1.000000000000000000 ) ) ;
#7710=CYLINDRICAL_SURFACE ( 'NONE', #3133, 15.00000000000000000 ) ;
#7750=CIRCLE ( 'NONE', #13466, 1.500000000000000666 ) ;
#7757=AXIS2_PLACEMENT_3D ( 'NONE', #2306, #5504, #3286 ) ;
#7774=ORIENTED_EDGE ( 'NONE', *, *, #2577, .F. ) ;
#7778=PRODUCT ( 'driver roller', 'driver roller', '', ( #11218 ) ) ;
#7795=EDGE_CURVE ( 'NONE', #1508, #3673, #6883, .T. ) ;
#7804=DIRECTION ( 'NONE',  ( -0.000000000000000000, -0.000000000000000000, -1.000000000000000000 ) ) ;
#7817=DIRECTION ( 'NONE',  ( -0.8660254037844412611, 0.4999999999999956146, 0.000000000000000000 ) ) ;
#7826=VERTEX_POINT ( 'NONE', #4872 ) ;
#7827=ORIENTED_EDGE ( 'NONE', *, *, #12563, .F. ) ;
#7829=CYLINDRICAL_SURFACE ( 'NONE', #348, 15.00000000000000000 ) ;
#7839=FACE_OUTER_BOUND ( 'NONE', #13450, .T. ) ;
#7866=CARTESIAN_POINT ( 'NONE',  ( 1.498123826657866475, -5.075000000000000178, 0.000000000000000000 ) ) ;
#7868=ADVANCED_FACE ( 'NONE', ( #11217 ), #12259, .F. ) ;
#7884=EDGE_CURVE ( 'NONE', #12293, #2807, #10528, .T. ) ;
#7896=AXIS2_PLACEMENT_3D ( 'NONE', #7153, #6394, #7223 ) ;
#7904=CYLINDRICAL_SURFACE ( 'NONE', #9323, 1.500000000000001332 ) ;
#7908=DIRECTION ( 'NONE',  ( -0.000000000000000000, -0.000000000000000000, -1.000000000000000000 ) ) ;
#7917=CYLINDRICAL_SURFACE ( 'NONE', #6556, 5.000000000000000888 ) ;
#7924=ORIENTED_EDGE ( 'NONE', *, *, #13033, .T. ) ;
#7937=VECTOR ( 'NONE', #12738, 1000.000000000000000 ) ;
#7940=EDGE_LOOP ( 'NONE', ( #4121, #1100, #9940, #9186 ) ) ;
#7952=VECTOR ( 'NONE', #5933, 1000.000000000000000 ) ;
#7957=ORIENTED_EDGE ( 'NONE', *, *, #8609, .T. ) ;
#7984=DIRECTION ( 'NONE',  ( 0.000000000000000000, 0.000000000000000000, 1.000000000000000000 ) ) ;
#7990=ORIENTED_EDGE ( 'NONE', *, *, #9483, .F. ) ;
#7995=ORIENTED_EDGE ( 'NONE', *, *, #846, .T. ) ;
#8008=ADVANCED_FACE ( 'NONE', ( #12602, #5428 ), #9364, .T. ) ;
#8011=ORIENTED_EDGE ( 'NONE', *, *, #13238, .F. ) ;
#8018=AXIS2_PLACEMENT_3D ( 'NONE', #11898, #9830, #349 ) ;
#8036=ADVANCED_FACE ( 'NONE', ( #153 ), #11636, .T. ) ;
#8058=AXIS2_PLACEMENT_3D ( 'NONE', #5604, #4559, #9612 ) ;
#8066=ORIENTED_EDGE ( 'NONE', *, *, #11077, .F. ) ;
#8072=EDGE_CURVE ( 'NONE', #2996, #4555, #8794, .T. ) ;
#8075=LINE ( 'NONE', #1622, #5320 ) ;
#8088=ADVANCED_FACE ( 'NONE', ( #3612 ), #2563, .F. ) ;
#8091=AXIS2_PLACEMENT_3D ( 'NONE', #9625, #2418, #151 ) ;
#8097=ORIENTED_EDGE ( 'NONE', *, *, #12695, .T. ) ;
#8101=DIRECTION ( 'NONE',  ( 0.000000000000000000, 0.000000000000000000, 1.000000000000000000 ) ) ;
#8115=ORIENTED_EDGE ( 'NONE', *, *, #12563, .T. ) ;
#8120=DIRECTION ( 'NONE',  ( -1.000000000000000000, 0.000000000000000000, 0.000000000000000000 ) ) ;
#8125=DIRECTION ( 'NONE',  ( -0.000000000000000000, -0.000000000000000000, -1.000000000000000000 ) ) ;
#8126=CARTESIAN_POINT ( 'NONE',  ( -13.67449106481169530, -13.83491329190050578, -9.000000000000000000 ) ) ;
#8129=DIRECTION ( 'NONE',  ( 0.000000000000000000, 0.000000000000000000, 1.000000000000000000 ) ) ;
#8151=EDGE_LOOP ( 'NONE', ( #3654, #9873, #3451, #896 ) ) ;
#8153=ORIENTED_EDGE ( 'NONE', *, *, #11191, .F. ) ;
#8170=CARTESIAN_POINT ( 'NONE',  ( 12.99038105676649835, -12.49999999999984901, 9.000000000000000000 ) ) ;
#8184=AXIS2_PLACEMENT_3D ( 'NONE', #7649, #10619, #5574 ) ;
#8201=DIRECTION ( 'NONE',  ( -0.4999999999999924505, -0.8660254037844429265, 0.000000000000000000 ) ) ;
#8206=DIRECTION ( 'NONE',  ( 1.000000000000000000, 0.000000000000000000, 0.000000000000000000 ) ) ;
#8254=EDGE_LOOP ( 'NONE', ( #951, #11605, #4763, #10408 ) ) ;
#8278=DIRECTION ( 'NONE',  ( -0.8660254037844412611, 0.4999999999999956146, 0.000000000000000000 ) ) ;
#8282=CARTESIAN_POINT ( 'NONE',  ( -6.000000000000012434, -7.009618943233427935, -9.000000000000000000 ) ) ;
#8283=AXIS2_PLACEMENT_3D ( 'NONE', #5015, #5984, #1667 ) ;
#8284=CARTESIAN_POINT ( 'NONE',  ( 6.165086708099646984, -33.67449106481162602, -9.000000000000000000 ) ) ;
#8326=ORIENTED_EDGE ( 'NONE', *, *, #7884, .F. ) ;
#8331=CARTESIAN_POINT ( 'NONE',  ( 15.00000000000000355, -19.99999999999984368, 9.000000000000000000 ) ) ;
#8387=EDGE_CURVE ( 'NONE', #6599, #1223, #7750, .T. ) ;
#8389=ORIENTED_EDGE ( 'NONE', *, *, #11991, .T. ) ;
#8393=AXIS2_PLACEMENT_3D ( 'NONE', #4563, #8782, #6714 ) ;
#8401=EDGE_CURVE ( 'NONE', #6266, #3891, #9514, .T. ) ;
#8403=DIRECTION ( 'NONE',  ( 0.000000000000000000, -0.000000000000000000, 1.000000000000000000 ) ) ;
#8435=CARTESIAN_POINT ( 'NONE',  ( 8.759913291900563337, -32.17636723815374467, 0.000000000000000000 ) ) ;
#8439=ORIENTED_EDGE ( 'NONE', *, *, #7884, .T. ) ;
#8451=CIRCLE ( 'NONE', #9778, 1.500000000000001110 ) ;
#8472=VERTEX_POINT ( 'NONE', #3946 ) ;
#8473=EDGE_CURVE ( 'NONE', #10472, #3498, #9070, .T. ) ;
#8485=VECTOR ( 'NONE', #6481, 1000.000000000000000 ) ;
#8502=CARTESIAN_POINT ( 'NONE',  ( -7.499999999999923617, -32.99038105676662269, 9.000000000000000000 ) ) ;
#8526=DIRECTION ( 'NONE',  ( 0.000000000000000000, 0.000000000000000000, 1.000000000000000000 ) ) ;
#8551=LINE ( 'NONE', #4532, #49 ) ;
#8553=CARTESIAN_POINT ( 'NONE',  ( 2.449293598294706513E-15, -20.00000000000000000, -9.000000000000000000 ) ) ;
#8555=PLANE ( 'NONE',  #2485 ) ;
#8556=ORIENTED_EDGE ( 'NONE', *, *, #13348, .T. ) ;
#8583=ORIENTED_EDGE ( 'NONE', *, *, #5956, .F. ) ;
#8607=ORIENTED_EDGE ( 'NONE', *, *, #5014, .T. ) ;
#8609=EDGE_CURVE ( 'NONE', #10938, #4659, #12844, .T. ) ;
#8618=DIRECTION ( 'NONE',  ( 0.000000000000000000, 0.000000000000000000, -1.000000000000000000 ) ) ;
#8624=EDGE_LOOP ( 'NONE', ( #1439, #8153, #1033, #2733 ) ) ;
#8640=ORIENTED_EDGE ( 'NONE', *, *, #12523, .F. ) ;
#8655=CIRCLE ( 'NONE', #2025, 1.500000000000000222 ) ;
#8698=DIRECTION ( 'NONE',  ( 0.5000000000000103251, -0.8660254037844327124, 0.000000000000000000 ) ) ;
#8705=DIRECTION ( 'NONE',  ( -0.000000000000000000, -0.000000000000000000, -1.000000000000000000 ) ) ;
#8717=EDGE_CURVE ( 'NONE', #3891, #10160, #7540, .T. ) ;
#8722=EDGE_CURVE ( 'NONE', #1223, #2588, #10714, .T. ) ;
#8731=VECTOR ( 'NONE', #5394, 1000.000000000000000 ) ;
#8746=CARTESIAN_POINT ( 'NONE',  ( -7.500000000000013323, -7.009618943233427935, -9.000000000000000000 ) ) ;
#8750=DIRECTION ( 'NONE',  ( -1.000000000000000000, 0.000000000000000000, 0.000000000000000000 ) ) ;
#8765=SURFACE_STYLE_FILL_AREA ( #9346 ) ;
#8774=ORIENTED_EDGE ( 'NONE', *, *, #6846, .T. ) ;
#8777=ORIENTED_EDGE ( 'NONE', *, *, #6544, .F. ) ;
#8779=EDGE_CURVE ( 'NONE', #940, #6987, #2336, .T. ) ;
#8782=DIRECTION ( 'NONE',  ( 0.000000000000000000, 0.000000000000000000, 1.000000000000000000 ) ) ;
#8794=LINE ( 'NONE', #6591, #10634 ) ;
#8800=DIRECTION ( 'NONE',  ( -3.469446951953611033E-15, 1.000000000000000000, 0.000000000000000000 ) ) ;
#8829=FACE_OUTER_BOUND ( 'NONE', #7192, .T. ) ;
#8845=EDGE_LOOP ( 'NONE', ( #13278, #3603, #5922, #11824 ) ) ;
#8846=ORIENTED_EDGE ( 'NONE', *, *, #13238, .T. ) ;
#8882=AXIS2_PLACEMENT_3D ( 'NONE', #2956, #9517, #7324 ) ;
#8895=CIRCLE ( 'NONE', #1145, 1.499999999999998446 ) ;
#8897=ADVANCED_FACE ( 'NONE', ( #3929 ), #3658, .F. ) ;
#8927=CIRCLE ( 'NONE', #12449, 1.500000000000000666 ) ;
#8930=ORIENTED_EDGE ( 'NONE', *, *, #2362, .F. ) ;
#8931=VERTEX_POINT ( 'NONE', #7260 ) ;
#8940=VECTOR ( 'NONE', #11300, 1000.000000000000000 ) ;
#8942=CARTESIAN_POINT ( 'NONE',  ( -14.99999999999999645, -20.00000000000005329, -9.000000000000000000 ) ) ;
#8952=CIRCLE ( 'NONE', #9587, 1.500000000000001332 ) ;
#8962=DIRECTION ( 'NONE',  ( 0.000000000000000000, 0.000000000000000000, 1.000000000000000000 ) ) ;
#8990=EDGE_LOOP ( 'NONE', ( #6722, #3521, #2080, #10785 ) ) ;
#8998=CARTESIAN_POINT ( 'NONE',  ( -13.67449106481168997, -13.83491329190049690, 0.000000000000000000 ) ) ;
#9061=EDGE_CURVE ( 'NONE', #1857, #2067, #2091, .T. ) ;
#9067=AXIS2_PLACEMENT_3D ( 'NONE', #15, #4237, #6397 ) ;
#9069=CARTESIAN_POINT ( 'NONE',  ( 12.17636723815371447, -11.24008670809939581, 0.000000000000000000 ) ) ;
#9070=LINE ( 'NONE', #12309, #12153 ) ;
#9121=AXIS2_PLACEMENT_3D ( 'NONE', #5629, #3343, #3211 ) ;
#9154=CARTESIAN_POINT ( 'NONE',  ( 1.000000000000000000, -14.00000000000000000, -9.000000000000001776 ) ) ;
#9161=EDGE_CURVE ( 'NONE', #5207, #6478, #2631, .T. ) ;
#9172=ORIENTED_EDGE ( 'NONE', *, *, #6407, .F. ) ;
#9177=( LENGTH_UNIT ( ) NAMED_UNIT ( * ) SI_UNIT ( .MILLI., .METRE. ) );
#9186=ORIENTED_EDGE ( 'NONE', *, *, #10321, .F. ) ;
#9192=AXIS2_PLACEMENT_3D ( 'NONE', #5232, #7088, #10535 ) ;
#9194=CIRCLE ( 'NONE', #8091, 1.499999999999999334 ) ;
#9219=ORIENTED_EDGE ( 'NONE', *, *, #7136, .F. ) ;
#9234=EDGE_CURVE ( 'NONE', #1857, #2807, #4857, .T. ) ;
#9235=ORIENTED_EDGE ( 'NONE', *, *, #6947, .T. ) ;
#9239=CARTESIAN_POINT ( 'NONE',  ( 2.449293598294706513E-15, -20.00000000000000000, 9.000000000000000000 ) ) ;
#9252=ORIENTED_EDGE ( 'NONE', *, *, #13369, .F. ) ;
#9254=CIRCLE ( 'NONE', #11236, 15.00000000000000000 ) ;
#9264=AXIS2_PLACEMENT_3D ( 'NONE', #4381, #11146, #1665 ) ;
#9299=DIRECTION ( 'NONE',  ( 0.000000000000000000, 1.000000000000000000, 0.000000000000000000 ) ) ;
#9306=CARTESIAN_POINT ( 'NONE',  ( 1.498123826657866253, -34.92499999999999716, 9.000000000000000000 ) ) ;
#9323=AXIS2_PLACEMENT_3D ( 'NONE', #2065, #6863, #12114 ) ;
#9346=FILL_AREA_STYLE ('',( #1273 ) ) ;
#9355=CARTESIAN_POINT ( 'NONE',  ( -7.500000000000013323, -7.009618943233427935, 9.000000000000000000 ) ) ;
#9364=PLANE ( 'NONE',  #1121 ) ;
#9374=CIRCLE ( 'NONE', #4082, 1.500000000000001332 ) ;
#9377=VERTEX_POINT ( 'NONE', #803 ) ;
#9447=LINE ( 'NONE', #11532, #7076 ) ;
#9449=DIRECTION ( 'NONE',  ( 0.000000000000000000, 0.000000000000000000, 1.000000000000000000 ) ) ;
#9450=CARTESIAN_POINT ( 'NONE',  ( 2.449293598294706513E-15, -20.00000000000000000, -9.000000000000000000 ) ) ;
#9470=AXIS2_PLACEMENT_3D ( 'NONE', #9239, #13297, #7171 ) ;
#9483=EDGE_CURVE ( 'NONE', #6478, #2588, #5747, .T. ) ;
#9491=DIRECTION ( 'NONE',  ( 1.000000000000000000, 0.000000000000000000, 0.000000000000000000 ) ) ;
#9492=CARTESIAN_POINT ( 'NONE',  ( -11.49038105676654453, -27.50000000000006040, -9.000000000000000000 ) ) ;
#9499=EDGE_CURVE ( 'NONE', #6494, #11878, #9533, .T. ) ;
#9502=STYLED_ITEM ( 'NONE', ( #11559 ), #11781 ) ;
#9505=CARTESIAN_POINT ( 'NONE',  ( -12.17636723815382993, -11.24008670809956456, 9.000000000000000000 ) ) ;
#9514=CIRCLE ( 'NONE', #12, 1.500000000000001110 ) ;
#9517=DIRECTION ( 'NONE',  ( 0.000000000000000000, 0.000000000000000000, 1.000000000000000000 ) ) ;
#9518=DIRECTION ( 'NONE',  ( 1.000000000000000000, 0.000000000000000000, 0.000000000000000000 ) ) ;
#9528=CARTESIAN_POINT ( 'NONE',  ( 1.000000000000000000, -14.00000000000000000, 8.999999999999998224 ) ) ;
#9533=LINE ( 'NONE', #8435, #11490 ) ;
#9540=CIRCLE ( 'NONE', #3364, 1.500000000000000222 ) ;
#9542=ADVANCED_FACE ( 'NONE', ( #10565 ), #5198, .F. ) ;
#9546=CARTESIAN_POINT ( 'NONE',  ( -1.498123826657861368, -34.92499999999999716, 9.000000000000000000 ) ) ;
#9553=ORIENTED_EDGE ( 'NONE', *, *, #272, .F. ) ;
#9584=EDGE_CURVE ( 'NONE', #9377, #4470, #12143, .T. ) ;
#9587=AXIS2_PLACEMENT_3D ( 'NONE', #12759, #3303, #7526 ) ;
#9597=CIRCLE ( 'NONE', #12231, 1.500000000000000222 ) ;
#9608=EDGE_CURVE ( 'NONE', #12388, #6557, #2393, .T. ) ;
#9612=DIRECTION ( 'NONE',  ( -1.000000000000000000, 0.000000000000000000, 0.000000000000000000 ) ) ;
#9625=CARTESIAN_POINT ( 'NONE',  ( -12.99038105676654453, -27.50000000000006040, -9.000000000000000000 ) ) ;
#9647=DIRECTION ( 'NONE',  ( -0.000000000000000000, -0.000000000000000000, -1.000000000000000000 ) ) ;
#9654=CARTESIAN_POINT ( 'NONE',  ( 2.449293598294706513E-15, -20.00000000000000000, 9.000000000000000000 ) ) ;
#9662=DIRECTION ( 'NONE',  ( 1.000000000000000000, 0.000000000000000000, 0.000000000000000000 ) ) ;
#9673=VERTEX_POINT ( 'NONE', #4414 ) ;
#9675=DIRECTION ( 'NONE',  ( 1.000000000000000000, 0.000000000000000000, 0.000000000000000000 ) ) ;
#9710=MECHANICAL_DESIGN_GEOMETRIC_PRESENTATION_REPRESENTATION('',(#5975),#13532);
#9721=DIRECTION ( 'NONE',  ( 0.000000000000000000, 0.000000000000000000, 1.000000000000000000 ) ) ;
#9765=DIRECTION ( 'NONE',  ( -0.000000000000000000, -0.000000000000000000, -1.000000000000000000 ) ) ;
#9778=AXIS2_PLACEMENT_3D ( 'NONE', #2342, #6580, #4 ) ;
#9792=EDGE_CURVE ( 'NONE', #6392, #10628, #575, .T. ) ;
#9795=CARTESIAN_POINT ( 'NONE',  ( -7.500000000000013323, -7.009618943233427935, -9.000000000000000000 ) ) ;
#9796=ADVANCED_FACE ( 'NONE', ( #2670 ), #11104, .F. ) ;
#9825=EDGE_CURVE ( 'NONE', #4959, #7079, #8075, .T. ) ;
#9827=EDGE_CURVE ( 'NONE', #7673, #7674, #10207, .T. ) ;
#9830=DIRECTION ( 'NONE',  ( 0.000000000000000000, 0.000000000000000000, 1.000000000000000000 ) ) ;
#9833=FACE_OUTER_BOUND ( 'NONE', #3840, .T. ) ;
#9837=PLANE ( 'NONE',  #6674 ) ;
#9843=ORIENTED_EDGE ( 'NONE', *, *, #13608, .T. ) ;
#9845=CARTESIAN_POINT ( 'NONE',  ( 2.449293598294706513E-15, -35.00000000000000000, -9.000000000000000000 ) ) ;
#9862=FACE_OUTER_BOUND ( 'NONE', #4813, .T. ) ;
#9873=ORIENTED_EDGE ( 'NONE', *, *, #11405, .T. ) ;
#9908=DIRECTION ( 'NONE',  ( -0.000000000000000000, 0.000000000000000000, 1.000000000000000000 ) ) ;
#9919=UNCERTAINTY_MEASURE_WITH_UNIT (LENGTH_MEASURE( 1.000000000000000082E-05 ), #10825, 'distance_accuracy_value', 'NONE');
#9928=ADVANCED_FACE ( 'NONE', ( #11595 ), #13646, .T. ) ;
#9936=CIRCLE ( 'NONE', #8184, 1.499999999999998446 ) ;
#9940=ORIENTED_EDGE ( 'NONE', *, *, #12212, .T. ) ;
#9951=EDGE_CURVE ( 'NONE', #278, #13382, #9447, .T. ) ;
#9959=EDGE_CURVE ( 'NONE', #5207, #1369, #11028, .T. ) ;
#9983=ORIENTED_EDGE ( 'NONE', *, *, #9584, .F. ) ;
#10002=ORIENTED_EDGE ( 'NONE', *, *, #3284, .F. ) ;
#10020=VERTEX_POINT ( 'NONE', #8284 ) ;
#10025=CIRCLE ( 'NONE', #7177, 15.00000000000000000 ) ;
#10051=ORIENTED_EDGE ( 'NONE', *, *, #8387, .T. ) ;
#10054=CARTESIAN_POINT ( 'NONE',  ( 12.17636723815389566, -28.75991329190035373, -9.000000000000000000 ) ) ;
#10060=ADVANCED_FACE ( 'NONE', ( #6485 ), #6549, .T. ) ;
#10068=CIRCLE ( 'NONE', #9192, 1.500000000000001332 ) ;
#10069=EDGE_CURVE ( 'NONE', #11878, #10020, #9936, .T. ) ;
#10071=VECTOR ( 'NONE', #4719, 1000.000000000000000 ) ;
#10109=DIRECTION ( 'NONE',  ( 1.000000000000000000, 0.000000000000000000, 0.000000000000000000 ) ) ;
#10119=LINE ( 'NONE', #631, #8940 ) ;
#10121=AXIS2_PLACEMENT_3D ( 'NONE', #8170, #2983, #4151 ) ;
#10129=DIRECTION ( 'NONE',  ( 0.000000000000000000, 0.000000000000000000, 1.000000000000000000 ) ) ;
#10157=DIRECTION ( 'NONE',  ( 0.4999999999999977796, 0.8660254037844398178, 0.000000000000000000 ) ) ;
#10160=VERTEX_POINT ( 'NONE', #7225 ) ;
#10185=DIRECTION ( 'NONE',  ( 0.000000000000000000, 0.000000000000000000, 1.000000000000000000 ) ) ;
#10187=AXIS2_PLACEMENT_3D ( 'NONE', #5587, #317, #12008 ) ;
#10207=LINE ( 'NONE', #7031, #7952 ) ;
#10216=ORIENTED_EDGE ( 'NONE', *, *, #9061, .F. ) ;
#10235=CARTESIAN_POINT ( 'NONE',  ( -7.499999999999923617, -32.99038105676662269, -9.000000000000000000 ) ) ;
#10249=CIRCLE ( 'NONE', #6082, 15.00000000000000000 ) ;
#10250=ORIENTED_EDGE ( 'NONE', *, *, #12523, .T. ) ;
#10254=CARTESIAN_POINT ( 'NONE',  ( -14.99999999999999645, -20.00000000000005329, -9.000000000000000000 ) ) ;
#10261=FACE_OUTER_BOUND ( 'NONE', #6990, .T. ) ;
#10268=VERTEX_POINT ( 'NONE', #5690 ) ;
#10271=FACE_OUTER_BOUND ( 'NONE', #1943, .T. ) ;
#10275=DIRECTION ( 'NONE',  ( -1.000000000000000000, 0.000000000000000000, 0.000000000000000000 ) ) ;
#10278=DIRECTION ( 'NONE',  ( 1.000000000000000000, 0.000000000000000000, 0.000000000000000000 ) ) ;
#10319=CARTESIAN_POINT ( 'NONE',  ( -12.99038105676659427, -12.50000000000003020, -9.000000000000000000 ) ) ;
#10321=EDGE_CURVE ( 'NONE', #11056, #8472, #3810, .T. ) ;
#10324=ADVANCED_FACE ( 'NONE', ( #12240 ), #1792, .T. ) ;
#10361=DIRECTION ( 'NONE',  ( 1.000000000000000000, 0.000000000000000000, 0.000000000000000000 ) ) ;
#10407=ORIENTED_EDGE ( 'NONE', *, *, #13564, .F. ) ;
#10408=ORIENTED_EDGE ( 'NONE', *, *, #1220, .F. ) ;
#10415=FACE_BOUND ( 'NONE', #2038, .T. ) ;
#10416=DIRECTION ( 'NONE',  ( 0.000000000000000000, 0.000000000000000000, 1.000000000000000000 ) ) ;
#10422=ADVANCED_FACE ( 'NONE', ( #5827 ), #744, .F. ) ;
#10444=( LENGTH_UNIT ( ) NAMED_UNIT ( * ) SI_UNIT ( .MILLI., .METRE. ) );
#10445=DIRECTION ( 'NONE',  ( 0.000000000000000000, -0.000000000000000000, 1.000000000000000000 ) ) ;
#10453=ORIENTED_EDGE ( 'NONE', *, *, #8401, .T. ) ;
#10455=EDGE_LOOP ( 'NONE', ( #5582, #392, #4487, #5961 ) ) ;
#10472=VERTEX_POINT ( 'NONE', #11130 ) ;
#10521=SHAPE_REPRESENTATION ( 'driver roller', ( #430 ), #13240 ) ;
#10523=ORIENTED_EDGE ( 'NONE', *, *, #5326, .F. ) ;
#10528=LINE ( 'NONE', #9492, #3570 ) ;
#10535=DIRECTION ( 'NONE',  ( -3.469446951953611033E-15, 1.000000000000000000, 0.000000000000000000 ) ) ;
#10539=CARTESIAN_POINT ( 'NONE',  ( -4.999999999999998224, -20.00000000000000000, 15.00000000000000355 ) ) ;
#10559=LINE ( 'NONE', #5518, #8731 ) ;
#10565=FACE_OUTER_BOUND ( 'NONE', #11729, .T. ) ;
#10589=ORIENTED_EDGE ( 'NONE', *, *, #7450, .T. ) ;
#10595=AXIS2_PLACEMENT_3D ( 'NONE', #3915, #13304, #10278 ) ;
#10607=AXIS2_PLACEMENT_3D ( 'NONE', #239, #9647, #8750 ) ;
#10614=FACE_OUTER_BOUND ( 'NONE', #6848, .T. ) ;
#10619=DIRECTION ( 'NONE',  ( 0.000000000000000000, 0.000000000000000000, 1.000000000000000000 ) ) ;
#10628=VERTEX_POINT ( 'NONE', #4830 ) ;
#10634=VECTOR ( 'NONE', #4718, 1000.000000000000000 ) ;
#10653=AXIS2_PLACEMENT_3D ( 'NONE', #5138, #4092, #3706 ) ;
#10659=ORIENTED_EDGE ( 'NONE', *, *, #4827, .F. ) ;
#10672=ADVANCED_FACE ( 'NONE', ( #2055 ), #4904, .F. ) ;
#10700=CARTESIAN_POINT ( 'NONE',  ( 2.449293598294706513E-15, -5.000000000000000888, -9.000000000000000000 ) ) ;
#10714=LINE ( 'NONE', #4560, #7321 ) ;
#10716=DIRECTION ( 'NONE',  ( 0.000000000000000000, 0.000000000000000000, 1.000000000000000000 ) ) ;
#10722=EDGE_LOOP ( 'NONE', ( #3383, #4364, #9983, #8640, #1926, #1969, #5317, #7672, #7990, #1249, #4591, #11797, #12317, #12320, #11379, #2503, #3483, #9252, #12872, #3317, #8389, #10659, #4795, #11444, #8846, #13004, #6642, #4497, #2345 ) ) ;
#10723=VERTEX_POINT ( 'NONE', #7113 ) ;
#10728=CARTESIAN_POINT ( 'NONE',  ( 2.449293598294706513E-15, -20.00000000000000000, 9.000000000000000000 ) ) ;
#10742=CARTESIAN_POINT ( 'NONE',  ( -8.759913291900485177, -7.823632761846201156, -9.000000000000000000 ) ) ;
#10761=SURFACE_SIDE_STYLE ('',( #8765 ) ) ;
#10774=DIRECTION ( 'NONE',  ( -0.000000000000000000, -0.000000000000000000, 1.000000000000000000 ) ) ;
#10785=ORIENTED_EDGE ( 'NONE', *, *, #7030, .T. ) ;
#10786=FACE_OUTER_BOUND ( 'NONE', #10984, .T. ) ;
#10794=DIRECTION ( 'NONE',  ( -1.000000000000000000, -4.082155997157843695E-16, 0.000000000000000000 ) ) ;
#10799=ORIENTED_EDGE ( 'NONE', *, *, #11947, .T. ) ;
#10806=LINE ( 'NONE', #6351, #8485 ) ;
#10825=( LENGTH_UNIT ( ) NAMED_UNIT ( * ) SI_UNIT ( .MILLI., .METRE. ) );
#10839=ORIENTED_EDGE ( 'NONE', *, *, #10069, .F. ) ;
#10850=AXIS2_PLACEMENT_3D ( 'NONE', #3961, #7081, #1740 ) ;
#10852=CIRCLE ( 'NONE', #4124, 1.500000000000000666 ) ;
#10856=ORIENTED_EDGE ( 'NONE', *, *, #12531, .F. ) ;
#10857=CARTESIAN_POINT ( 'NONE',  ( 1.000000000000000444, -15.10102051443364246, -8.999999999999998224 ) ) ;
#10884=DIRECTION ( 'NONE',  ( 4.082155997157843695E-16, -1.000000000000000000, 0.000000000000000000 ) ) ;
#10889=LINE ( 'NONE', #10958, #6173 ) ;
#10893=CARTESIAN_POINT ( 'NONE',  ( -12.17636723815376953, -28.75991329190052781, -9.000000000000000000 ) ) ;
#10923=EDGE_LOOP ( 'NONE', ( #11645, #3717, #11214, #5099 ) ) ;
#10938=VERTEX_POINT ( 'NONE', #6818 ) ;
#10943=EDGE_CURVE ( 'NONE', #9673, #4300, #1955, .T. ) ;
#10944=CARTESIAN_POINT ( 'NONE',  ( 2.449293598294706513E-15, -20.00000000000000000, 9.000000000000000000 ) ) ;
#10958=CARTESIAN_POINT ( 'NONE',  ( -0.9999999999999976685, -20.00000000000000000, -9.000000000000001776 ) ) ;
#10966=ADVANCED_FACE ( 'NONE', ( #8829 ), #5793, .F. ) ;
#10976=DIRECTION ( 'NONE',  ( 0.000000000000000000, -0.000000000000000000, 1.000000000000000000 ) ) ;
#10984=EDGE_LOOP ( 'NONE', ( #1755, #2712, #5533, #13415 ) ) ;
#10988=DIRECTION ( 'NONE',  ( -0.000000000000000000, -0.000000000000000000, -1.000000000000000000 ) ) ;
#10990=DIRECTION ( 'NONE',  ( 0.000000000000000000, 0.000000000000000000, 1.000000000000000000 ) ) ;
#10991=DIRECTION ( 'NONE',  ( -0.000000000000000000, 0.000000000000000000, 1.000000000000000000 ) ) ;
#11003=ORIENTED_EDGE ( 'NONE', *, *, #4329, .T. ) ;
#11019=AXIS2_PLACEMENT_3D ( 'NONE', #4634, #10716, #7817 ) ;
#11028=CIRCLE ( 'NONE', #2877, 15.00000000000000000 ) ;
#11029=CARTESIAN_POINT ( 'NONE',  ( 7.500000000000107470, -32.99038105676652322, 9.000000000000000000 ) ) ;
#11055=CIRCLE ( 'NONE', #7757, 15.00000000000000000 ) ;
#11056=VERTEX_POINT ( 'NONE', #10054 ) ;
#11066=AXIS2_PLACEMENT_3D ( 'NONE', #1353, #8705, #4351 ) ;
#11075=AXIS2_PLACEMENT_3D ( 'NONE', #7663, #4475, #8698 ) ;
#11077=EDGE_CURVE ( 'NONE', #6557, #7826, #10889, .T. ) ;
#11079=DIRECTION ( 'NONE',  ( 1.000000000000000000, 0.000000000000000000, 0.000000000000000000 ) ) ;
#11080=EDGE_CURVE ( 'NONE', #7826, #13382, #5655, .T. ) ;
#11104=CYLINDRICAL_SURFACE ( 'NONE', #10595, 1.500000000000001332 ) ;
#11114=ADVANCED_FACE ( 'NONE', ( #10271 ), #7243, .T. ) ;
#11128=EDGE_LOOP ( 'NONE', ( #5755, #4203, #7571, #5924 ) ) ;
#11130=CARTESIAN_POINT ( 'NONE',  ( 13.67449106481161003, -13.83491329190030861, -9.000000000000000000 ) ) ;
#11139=FACE_OUTER_BOUND ( 'NONE', #8990, .T. ) ;
#11146=DIRECTION ( 'NONE',  ( 0.000000000000000000, 0.000000000000000000, 1.000000000000000000 ) ) ;
#11148=ORIENTED_EDGE ( 'NONE', *, *, #9825, .F. ) ;
#11160=CARTESIAN_POINT ( 'NONE',  ( -6.165086708099442703, -33.67449106481171839, -9.000000000000000000 ) ) ;
#11177=VECTOR ( 'NONE', #13425, 1000.000000000000000 ) ;
#11191=EDGE_CURVE ( 'NONE', #4030, #6599, #4174, .T. ) ;
#11199=CARTESIAN_POINT ( 'NONE',  ( 12.99038105676665289, -27.49999999999988276, -9.000000000000000000 ) ) ;
#11203=LINE ( 'NONE', #478, #10071 ) ;
#11214=ORIENTED_EDGE ( 'NONE', *, *, #505, .T. ) ;
#11217=FACE_OUTER_BOUND ( 'NONE', #3873, .T. ) ;
#11218=PRODUCT_CONTEXT ( 'NONE', #12976, 'mechanical' ) ;
#11224=DIRECTION ( 'NONE',  ( 0.000000000000000000, 0.000000000000000000, 1.000000000000000000 ) ) ;
#11236=AXIS2_PLACEMENT_3D ( 'NONE', #8553, #3292, #9518 ) ;
#11238=CARTESIAN_POINT ( 'NONE',  ( 2.449293598294706513E-15, -20.00000000000000000, 9.000000000000000000 ) ) ;
#11241=( GEOMETRIC_REPRESENTATION_CONTEXT ( 3 ) GLOBAL_UNCERTAINTY_ASSIGNED_CONTEXT ( ( #9919 ) ) GLOBAL_UNIT_ASSIGNED_CONTEXT ( ( #10825, #318, #4474 ) ) REPRESENTATION_CONTEXT ( 'NONE', 'WORKASPACE' ) );
#11244=CARTESIAN_POINT ( 'NONE',  ( -13.49999999999999467, -20.00000000000005329, -9.000000000000000000 ) ) ;
#11252=PRODUCT_DEFINITION_FORMATION_WITH_SPECIFIED_SOURCE ( 'ANY', '', #7778, .NOT_KNOWN. ) ;
#11296=PLANE ( 'NONE',  #1900 ) ;
#11300=DIRECTION ( 'NONE',  ( 0.000000000000000000, -0.000000000000000000, -1.000000000000000000 ) ) ;
#11307=CARTESIAN_POINT ( 'NONE',  ( -1.000000000000000000, -14.00000000000000000, -9.000000000000001776 ) ) ;
#11308=DIRECTION ( 'NONE',  ( 1.000000000000000000, -6.938893903907227392E-16, 0.000000000000000000 ) ) ;
#11314=DIRECTION ( 'NONE',  ( 0.000000000000000000, -0.000000000000000000, 1.000000000000000000 ) ) ;
#11342=EDGE_CURVE ( 'NONE', #10268, #4657, #11676, .T. ) ;
#11364=DIRECTION ( 'NONE',  ( -0.000000000000000000, -0.000000000000000000, 1.000000000000000000 ) ) ;
#11379=ORIENTED_EDGE ( 'NONE', *, *, #3933, .T. ) ;
#11391=VERTEX_POINT ( 'NONE', #10742 ) ;
#11393=ORIENTED_EDGE ( 'NONE', *, *, #8779, .T. ) ;
#11405=EDGE_CURVE ( 'NONE', #6039, #4300, #1250, .T. ) ;
#11426=DIRECTION ( 'NONE',  ( 0.000000000000000000, 0.000000000000000000, 1.000000000000000000 ) ) ;
#11436=CYLINDRICAL_SURFACE ( 'NONE', #2555, 5.000000000000000888 ) ;
#11444=ORIENTED_EDGE ( 'NONE', *, *, #5014, .F. ) ;
#11458=ORIENTED_EDGE ( 'NONE', *, *, #7795, .F. ) ;
#11465=DIRECTION ( 'NONE',  ( 0.000000000000000000, 0.000000000000000000, 1.000000000000000000 ) ) ;
#11471=CIRCLE ( 'NONE', #850, 5.000000000000000888 ) ;
#11490=VECTOR ( 'NONE', #11549, 1000.000000000000000 ) ;
#11531=EDGE_CURVE ( 'NONE', #5893, #10938, #1968, .T. ) ;
#11532=CARTESIAN_POINT ( 'NONE',  ( 1.000000000000002442, -20.00000000000000000, -9.000000000000001776 ) ) ;
#11549=DIRECTION ( 'NONE',  ( 0.000000000000000000, -0.000000000000000000, -1.000000000000000000 ) ) ;
#11559=PRESENTATION_STYLE_ASSIGNMENT (( #5588 ) ) ;
#11570=ORIENTED_EDGE ( 'NONE', *, *, #8717, .F. ) ;
#11588=AXIS2_PLACEMENT_3D ( 'NONE', #3767, #6881, #12068 ) ;
#11595=FACE_OUTER_BOUND ( 'NONE', #11970, .T. ) ;
#11597=EDGE_CURVE ( 'NONE', #2116, #3498, #2847, .T. ) ;
#11604=ORIENTED_EDGE ( 'NONE', *, *, #6846, .F. ) ;
#11605=ORIENTED_EDGE ( 'NONE', *, *, #11077, .T. ) ;
#11636=CYLINDRICAL_SURFACE ( 'NONE', #2023, 15.00000000000000000 ) ;
#11644=LINE ( 'NONE', #10539, #11795 ) ;
#11645=ORIENTED_EDGE ( 'NONE', *, *, #11947, .F. ) ;
#11655=PLANE ( 'NONE',  #6315 ) ;
#11676=CIRCLE ( 'NONE', #11891, 15.00000000000000000 ) ;
#11687=DIRECTION ( 'NONE',  ( 1.000000000000000000, 0.000000000000000000, 0.000000000000000000 ) ) ;
#11694=VECTOR ( 'NONE', #7804, 1000.000000000000000 ) ;
#11729=EDGE_LOOP ( 'NONE', ( #11604, #8777, #5668, #3013 ) ) ;
#11750=DIRECTION ( 'NONE',  ( -0.000000000000000000, -0.000000000000000000, 1.000000000000000000 ) ) ;
#11762=ORIENTED_EDGE ( 'NONE', *, *, #3933, .F. ) ;
#11764=CIRCLE ( 'NONE', #8018, 15.00000000000000000 ) ;
#11779=ORIENTED_EDGE ( 'NONE', *, *, #505, .F. ) ;
#11780=DIRECTION ( 'NONE',  ( 0.000000000000000000, 0.000000000000000000, 1.000000000000000000 ) ) ;
#11781=ADVANCED_BREP_SHAPE_REPRESENTATION ( '', ( #961, #430 ), #13240 ) ;
#11782=CARTESIAN_POINT ( 'NONE',  ( 1.498123826657877133, -34.92499999999999716, -9.000000000000000000 ) ) ;
#11788=DIRECTION ( 'NONE',  ( -1.000000000000000000, 0.000000000000000000, 0.000000000000000000 ) ) ;
#11795=VECTOR ( 'NONE', #4047, 1000.000000000000000 ) ;
#11797=ORIENTED_EDGE ( 'NONE', *, *, #13608, .F. ) ;
#11800=CYLINDRICAL_SURFACE ( 'NONE', #746, 1.500000000000000666 ) ;
#11824=ORIENTED_EDGE ( 'NONE', *, *, #11405, .F. ) ;
#11836=CIRCLE ( 'NONE', #6119, 15.00000000000000000 ) ;
#11837=CARTESIAN_POINT ( 'NONE',  ( -14.92500000000000249, -18.50187617334218970, -9.000000000000000000 ) ) ;
#11877=ORIENTED_EDGE ( 'NONE', *, *, #1521, .F. ) ;
#11878=VERTEX_POINT ( 'NONE', #3319 ) ;
#11891=AXIS2_PLACEMENT_3D ( 'NONE', #6348, #11780, #102 ) ;
#11893=AXIS2_PLACEMENT_3D ( 'NONE', #9450, #10416, #13650 ) ;
#11898=CARTESIAN_POINT ( 'NONE',  ( 2.449293598294706513E-15, -20.00000000000000000, -9.000000000000000000 ) ) ;
#11923=CARTESIAN_POINT ( 'NONE',  ( -12.17636723815382993, -11.24008670809956456, -9.000000000000000000 ) ) ;
#11933=MECHANICAL_DESIGN_GEOMETRIC_PRESENTATION_REPRESENTATION('',(#9502),#11241);
#11947=EDGE_CURVE ( 'NONE', #3673, #8931, #12893, .T. ) ;
#11970=EDGE_LOOP ( 'NONE', ( #6458, #7957, #8011, #13158 ) ) ;
#11982=DIRECTION ( 'NONE',  ( 0.000000000000000000, 0.000000000000000000, 1.000000000000000000 ) ) ;
#11986=LINE ( 'NONE', #6738, #5075 ) ;
#11991=EDGE_CURVE ( 'NONE', #2116, #582, #1638, .T. ) ;
#11996=EDGE_CURVE ( 'NONE', #4959, #7826, #68, .T. ) ;
#12008=DIRECTION ( 'NONE',  ( 1.000000000000000000, 0.000000000000000000, 0.000000000000000000 ) ) ;
#12016=DIRECTION ( 'NONE',  ( -3.469446951953611033E-15, 1.000000000000000000, 0.000000000000000000 ) ) ;
#12043=AXIS2_PLACEMENT_3D ( 'NONE', #2875, #12277, #11308 ) ;
#12044=DIRECTION ( 'NONE',  ( -1.000000000000000000, 0.000000000000000000, 0.000000000000000000 ) ) ;
#12068=DIRECTION ( 'NONE',  ( 1.000000000000000000, 0.000000000000000000, 0.000000000000000000 ) ) ;
#12089=EDGE_CURVE ( 'NONE', #3673, #7167, #655, .T. ) ;
#12108=CARTESIAN_POINT ( 'NONE',  ( -12.99038105676659427, -12.50000000000003020, -9.000000000000000000 ) ) ;
#12114=DIRECTION ( 'NONE',  ( 1.000000000000000000, 0.000000000000000000, 0.000000000000000000 ) ) ;
#12143=CIRCLE ( 'NONE', #12792, 1.500000000000001332 ) ;
#12153=VECTOR ( 'NONE', #13612, 1000.000000000000000 ) ;
#12154=VERTEX_POINT ( 'NONE', #13045 ) ;
#12155=ORIENTED_EDGE ( 'NONE', *, *, #5857, .T. ) ;
#12169=ORIENTED_EDGE ( 'NONE', *, *, #7136, .T. ) ;
#12196=DIRECTION ( 'NONE',  ( 1.000000000000000000, 0.000000000000000000, 0.000000000000000000 ) ) ;
#12212=EDGE_CURVE ( 'NONE', #1302, #8472, #6312, .T. ) ;
#12231=AXIS2_PLACEMENT_3D ( 'NONE', #1530, #10185, #4036 ) ;
#12240=FACE_OUTER_BOUND ( 'NONE', #6939, .T. ) ;
#12243=CARTESIAN_POINT ( 'NONE',  ( -0.9999999999999995559, -15.10102051443364246, -8.999999999999998224 ) ) ;
#12259=CYLINDRICAL_SURFACE ( 'NONE', #904, 1.500000000000001332 ) ;
#12271=ORIENTED_EDGE ( 'NONE', *, *, #8387, .F. ) ;
#12277=DIRECTION ( 'NONE',  ( -0.000000000000000000, -0.000000000000000000, -1.000000000000000000 ) ) ;
#12293=VERTEX_POINT ( 'NONE', #4140 ) ;
#12300=CARTESIAN_POINT ( 'NONE',  ( -12.99038105676659427, -12.50000000000003020, 9.000000000000000000 ) ) ;
#12304=ORIENTED_EDGE ( 'NONE', *, *, #12089, .F. ) ;
#12309=CARTESIAN_POINT ( 'NONE',  ( 13.67449106481161003, -13.83491329190030861, 0.000000000000000000 ) ) ;
#12317=ORIENTED_EDGE ( 'NONE', *, *, #2433, .T. ) ;
#12319=LINE ( 'NONE', #487, #6633 ) ;
#12320=ORIENTED_EDGE ( 'NONE', *, *, #6947, .F. ) ;
#12336=ORIENTED_EDGE ( 'NONE', *, *, #5326, .T. ) ;
#12368=ADVANCED_FACE ( 'NONE', ( #5321 ), #11800, .F. ) ;
#12388=VERTEX_POINT ( 'NONE', #5586 ) ;
#12390=VERTEX_POINT ( 'NONE', #3171 ) ;
#12392=FACE_OUTER_BOUND ( 'NONE', #13260, .T. ) ;
#12447=EDGE_CURVE ( 'NONE', #9673, #11391, #10559, .T. ) ;
#12449=AXIS2_PLACEMENT_3D ( 'NONE', #9845, #6675, #6870 ) ;
#12462=CIRCLE ( 'NONE', #2078, 15.00000000000000000 ) ;
#12485=( NAMED_UNIT ( * ) PLANE_ANGLE_UNIT ( ) SI_UNIT ( $, .RADIAN. ) );
#12493=PRODUCT_DEFINITION ( 'UNKNOWN', '', #11252, #2926 ) ;
#12495=DIRECTION ( 'NONE',  ( 1.000000000000000000, 0.000000000000000000, 0.000000000000000000 ) ) ;
#12523=EDGE_CURVE ( 'NONE', #7673, #9377, #8952, .T. ) ;
#12529=ORIENTED_EDGE ( 'NONE', *, *, #7795, .T. ) ;
#12531=EDGE_CURVE ( 'NONE', #2384, #439, #3704, .T. ) ;
#12563=EDGE_CURVE ( 'NONE', #2067, #12293, #4315, .T. ) ;
#12570=DIRECTION ( 'NONE',  ( 0.000000000000000000, 0.000000000000000000, 1.000000000000000000 ) ) ;
#12595=ORIENTED_EDGE ( 'NONE', *, *, #13369, .T. ) ;
#12602=FACE_OUTER_BOUND ( 'NONE', #10722, .T. ) ;
#12629=AXIS2_PLACEMENT_3D ( 'NONE', #6060, #11364, #10109 ) ;
#12639=CIRCLE ( 'NONE', #935, 15.00000000000000000 ) ;
#12673=DIRECTION ( 'NONE',  ( 0.000000000000000000, 0.000000000000000000, 1.000000000000000000 ) ) ;
#12685=VECTOR ( 'NONE', #6979, 1000.000000000000000 ) ;
#12695=EDGE_CURVE ( 'NONE', #278, #7167, #2965, .T. ) ;
#12724=ORIENTED_EDGE ( 'NONE', *, *, #11996, .T. ) ;
#12728=DIRECTION ( 'NONE',  ( 1.000000000000000000, 0.000000000000000000, -0.000000000000000000 ) ) ;
#12733=DIRECTION ( 'NONE',  ( -1.000000000000000000, 0.000000000000000000, 0.000000000000000000 ) ) ;
#12737=ORIENTED_EDGE ( 'NONE', *, *, #9951, .F. ) ;
#12738=DIRECTION ( 'NONE',  ( 0.000000000000000000, 0.000000000000000000, -1.000000000000000000 ) ) ;
#12752=CARTESIAN_POINT ( 'NONE',  ( 1.000000000000002442, -20.00000000000000000, 8.999999999999998224 ) ) ;
#12759=CARTESIAN_POINT ( 'NONE',  ( -14.99999999999999645, -20.00000000000005329, 9.000000000000000000 ) ) ;
#12768=CARTESIAN_POINT ( 'NONE',  ( -0.9999999999999995559, -15.10102051443364246, 15.00000000000000355 ) ) ;
#12792=AXIS2_PLACEMENT_3D ( 'NONE', #6566, #4550, #12016 ) ;
#12815=CYLINDRICAL_SURFACE ( 'NONE', #6252, 5.000000000000000888 ) ;
#12844=LINE ( 'NONE', #3455, #3332 ) ;
#12859=EDGE_CURVE ( 'NONE', #1843, #2996, #4986, .T. ) ;
#12872=ORIENTED_EDGE ( 'NONE', *, *, #13336, .T. ) ;
#12890=ADVANCED_FACE ( 'NONE', ( #10614 ), #7444, .F. ) ;
#12893=CIRCLE ( 'NONE', #8058, 5.000000000000000888 ) ;
#12935=AXIS2_PLACEMENT_3D ( 'NONE', #10728, #411, #2286 ) ;
#12937=ORIENTED_EDGE ( 'NONE', *, *, #12447, .F. ) ;
#12948=CARTESIAN_POINT ( 'NONE',  ( 2.449293598294706513E-15, -20.00000000000000000, 15.00000000000000355 ) ) ;
#12955=ORIENTED_EDGE ( 'NONE', *, *, #689, .F. ) ;
#12959=SHAPE_REPRESENTATION_RELATIONSHIP ( 'NONE' , 'NONE' ,  #10521, #11781 ) ;
#12965=EDGE_CURVE ( 'NONE', #5207, #4030, #10806, .T. ) ;
#12976=APPLICATION_CONTEXT ( 'automotive_design' ) ;
#12977=AXIS2_PLACEMENT_3D ( 'NONE', #9795, #3574, #1407 ) ;
#12991=ORIENTED_EDGE ( 'NONE', *, *, #5591, .F. ) ;
#12997=CYLINDRICAL_SURFACE ( 'NONE', #12935, 15.00000000000000000 ) ;
#13004=ORIENTED_EDGE ( 'NONE', *, *, #3208, .F. ) ;
#13009=VERTEX_POINT ( 'NONE', #11782 ) ;
#13033=EDGE_CURVE ( 'NONE', #13009, #12154, #8927, .T. ) ;
#13039=CIRCLE ( 'NONE', #4907, 15.00000000000000000 ) ;
#13045=CARTESIAN_POINT ( 'NONE',  ( -1.498123826657861368, -34.92499999999999716, -9.000000000000000000 ) ) ;
#13046=AXIS2_PLACEMENT_3D ( 'NONE', #554, #5844, #8120 ) ;
#13063=CARTESIAN_POINT ( 'NONE',  ( 2.449293598294706513E-15, -20.00000000000000000, 9.000000000000000000 ) ) ;
#13073=DIRECTION ( 'NONE',  ( -0.000000000000000000, -0.000000000000000000, -1.000000000000000000 ) ) ;
#13102=AXIS2_PLACEMENT_3D ( 'NONE', #925, #3222, #1192 ) ;
#13111=VECTOR ( 'NONE', #2648, 1000.000000000000000 ) ;
#13158=ORIENTED_EDGE ( 'NONE', *, *, #12531, .T. ) ;
#13228=CARTESIAN_POINT ( 'NONE',  ( -13.49999999999999467, -20.00000000000005329, -9.000000000000000000 ) ) ;
#13238=EDGE_CURVE ( 'NONE', #2384, #4659, #5851, .T. ) ;
#13240=( GEOMETRIC_REPRESENTATION_CONTEXT ( 3 ) GLOBAL_UNCERTAINTY_ASSIGNED_CONTEXT ( ( #1608 ) ) GLOBAL_UNIT_ASSIGNED_CONTEXT ( ( #10444, #3440, #3372 ) ) REPRESENTATION_CONTEXT ( 'NONE', 'WORKASPACE' ) );
#13242=EDGE_CURVE ( 'NONE', #1508, #7079, #1460, .T. ) ;
#13260=EDGE_LOOP ( 'NONE', ( #11762, #7621, #4048, #213 ) ) ;
#13277=EDGE_CURVE ( 'NONE', #4104, #4218, #9597, .T. ) ;
#13278=ORIENTED_EDGE ( 'NONE', *, *, #6031, .F. ) ;
#13285=CYLINDRICAL_SURFACE ( 'NONE', #12629, 1.500000000000000666 ) ;
#13297=DIRECTION ( 'NONE',  ( -0.000000000000000000, -0.000000000000000000, -1.000000000000000000 ) ) ;
#13304=DIRECTION ( 'NONE',  ( -0.000000000000000000, -0.000000000000000000, 1.000000000000000000 ) ) ;
#13322=EDGE_LOOP ( 'NONE', ( #146, #10453, #13464, #10002, #4777, #13479, #8583, #7483, #261, #1234, #1645, #8774, #3959, #3198, #7075, #11003, #6771, #5841, #6783, #7924, #6124, #821, #10051, #10407, #8115, #3081, #5753, #12336, #5514 ) ) ;
#13323=CIRCLE ( 'NONE', #4744, 15.00000000000000000 ) ;
#13336=EDGE_CURVE ( 'NONE', #6392, #3498, #10025, .T. ) ;
#13348=EDGE_CURVE ( 'NONE', #2807, #6987, #6517, .T. ) ;
#13369=EDGE_CURVE ( 'NONE', #6392, #4555, #9374, .T. ) ;
#13371=( NAMED_UNIT ( * ) SI_UNIT ( $, .STERADIAN. ) SOLID_ANGLE_UNIT ( ) );
#13382=VERTEX_POINT ( 'NONE', #9154 ) ;
#13409=VERTEX_POINT ( 'NONE', #5909 ) ;
#13415=ORIENTED_EDGE ( 'NONE', *, *, #8473, .T. ) ;
#13417=FACE_OUTER_BOUND ( 'NONE', #1774, .T. ) ;
#13425=DIRECTION ( 'NONE',  ( 0.000000000000000000, -0.000000000000000000, 1.000000000000000000 ) ) ;
#13430=ORIENTED_EDGE ( 'NONE', *, *, #9827, .F. ) ;
#13437=DIRECTION ( 'NONE',  ( -0.000000000000000000, -0.000000000000000000, -1.000000000000000000 ) ) ;
#13440=CARTESIAN_POINT ( 'NONE',  ( 1.498123826657866475, -5.075000000000000178, 9.000000000000000000 ) ) ;
#13447=VERTEX_POINT ( 'NONE', #2857 ) ;
#13450=EDGE_LOOP ( 'NONE', ( #1898, #7093, #7311, #11393 ) ) ;
#13464=ORIENTED_EDGE ( 'NONE', *, *, #6031, .T. ) ;
#13466=AXIS2_PLACEMENT_3D ( 'NONE', #10235, #5968, #1582 ) ;
#13479=ORIENTED_EDGE ( 'NONE', *, *, #11531, .T. ) ;
#13484=DIRECTION ( 'NONE',  ( 1.000000000000000000, 0.000000000000000000, 0.000000000000000000 ) ) ;
#13486=DIRECTION ( 'NONE',  ( 1.000000000000000000, 0.000000000000000000, 0.000000000000000000 ) ) ;
#13493=FACE_OUTER_BOUND ( 'NONE', #2054, .T. ) ;
#13498=EDGE_LOOP ( 'NONE', ( #2452, #2381, #12155, #6602 ) ) ;
#13504=CARTESIAN_POINT ( 'NONE',  ( -7.499999999999923617, -32.99038105676662269, -9.000000000000000000 ) ) ;
#13518=AXIS2_PLACEMENT_3D ( 'NONE', #10319, #825, #13484 ) ;
#13532=( GEOMETRIC_REPRESENTATION_CONTEXT ( 3 ) GLOBAL_UNCERTAINTY_ASSIGNED_CONTEXT ( ( #5009 ) ) GLOBAL_UNIT_ASSIGNED_CONTEXT ( ( #9177, #12485, #13371 ) ) REPRESENTATION_CONTEXT ( 'NONE', 'WORKASPACE' ) );
#13562=DIRECTION ( 'NONE',  ( 0.000000000000000000, -0.000000000000000000, 1.000000000000000000 ) ) ;
#13564=EDGE_CURVE ( 'NONE', #2067, #1223, #6726, .T. ) ;
#13585=DIRECTION ( 'NONE',  ( 0.000000000000000000, 0.000000000000000000, 1.000000000000000000 ) ) ;
#13597=AXIS2_PLACEMENT_3D ( 'NONE', #772, #980, #2864 ) ;
#13606=EDGE_CURVE ( 'NONE', #7673, #6987, #10249, .T. ) ;
#13608=EDGE_CURVE ( 'NONE', #579, #1369, #7524, .T. ) ;
#13612=DIRECTION ( 'NONE',  ( -0.000000000000000000, -0.000000000000000000, 1.000000000000000000 ) ) ;
#13625=DIRECTION ( 'NONE',  ( 0.000000000000000000, 0.000000000000000000, 1.000000000000000000 ) ) ;
#13631=LINE ( 'NONE', #5090, #11177 ) ;
#13646=CYLINDRICAL_SURFACE ( 'NONE', #3315, 15.00000000000000000 ) ;
#13650=DIRECTION ( 'NONE',  ( 1.000000000000000000, 0.000000000000000000, 0.000000000000000000 ) ) ;
#13654=ORIENTED_EDGE ( 'NONE', *, *, #3208, .T. ) ;
#13658=DIRECTION ( 'NONE',  ( -0.4999999999999924505, -0.8660254037844429265, 0.000000000000000000 ) ) ;
#13662=AXIS2_PLACEMENT_3D ( 'NONE', #7402, #7467, #3035 ) ;
#13685=COLOUR_RGB('Light Blue',0.38,0.62,0.78);
#13686=FILL_AREA_STYLE_COLOUR('',#13685);
#13687=FILL_AREA_STYLE('',(#13686));
#13688=SURFACE_STYLE_FILL_AREA(#13687);
#13689=SURFACE_SIDE_STYLE('',(#13688));
#13690=SURFACE_STYLE_USAGE(.BOTH.,#13689);
#13691=PRESENTATION_STYLE_ASSIGNMENT((#13690));
ENDSEC;
END-ISO-10303-21;
